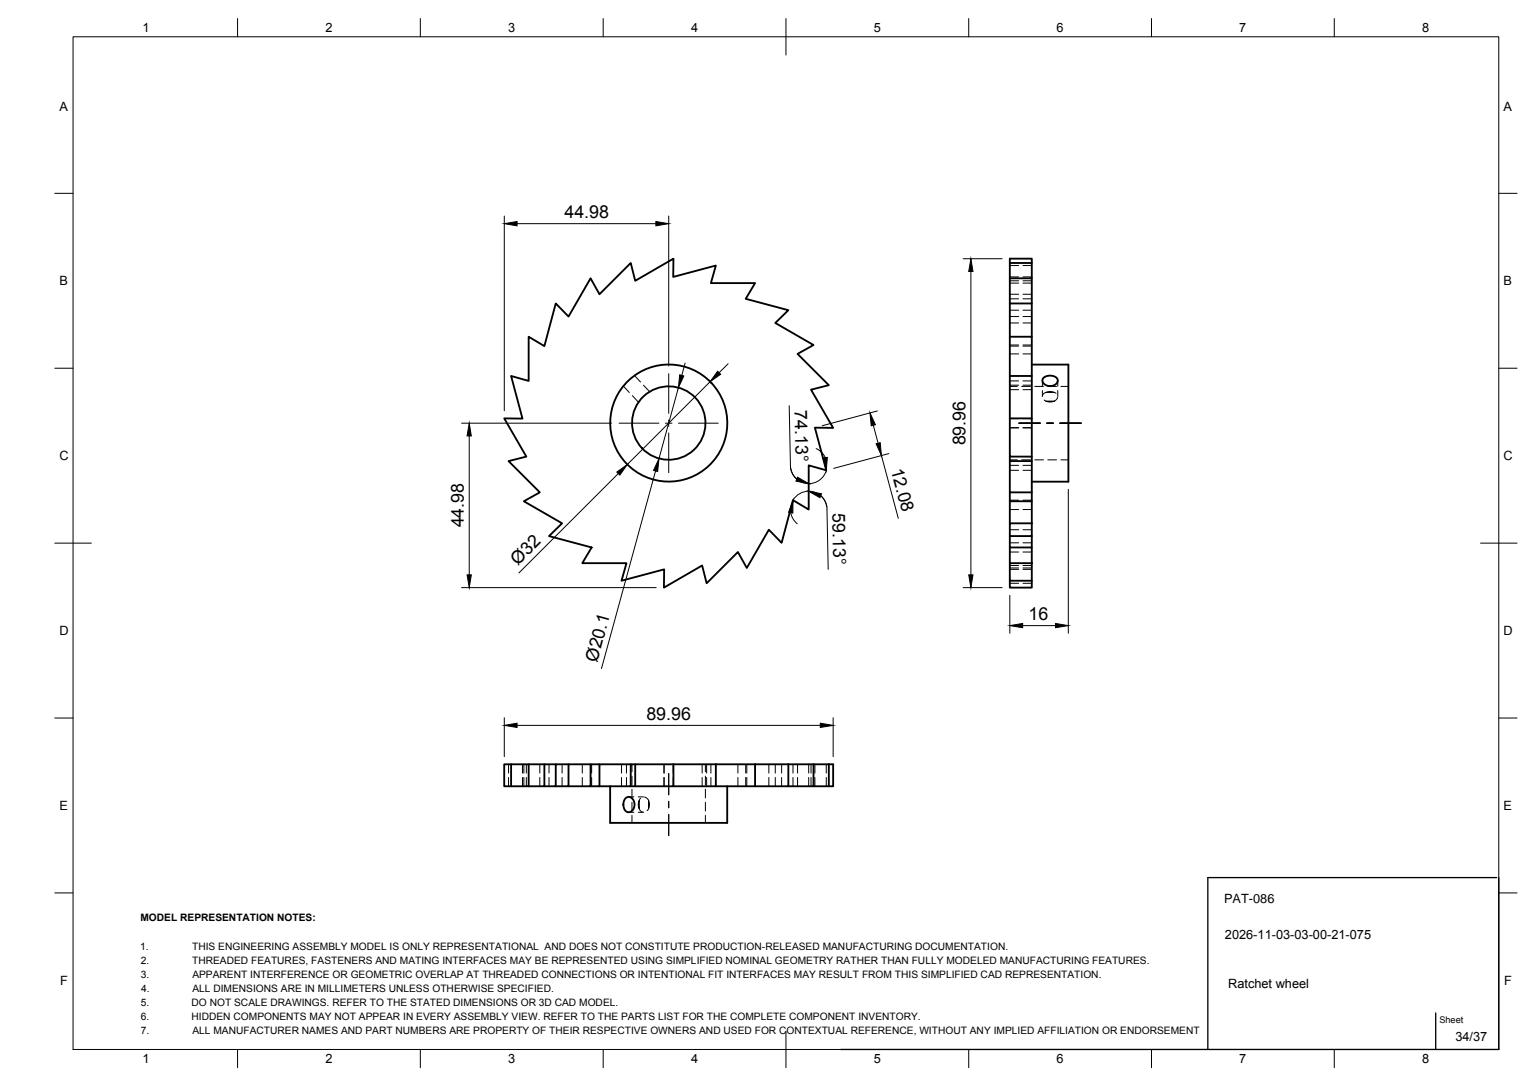
ISO-10303-21;
HEADER;
/* Generated by software containing ST-Developer
 * from STEP Tools, Inc. (www.steptools.com) 
 */

FILE_DESCRIPTION(
/* description */ ('Ratchet and pawl hand winch drum'),
/* implementation_level */ '2;1');

FILE_NAME(
/* name */ 'Ratchet wheel.step',
/* time_stamp */ '2026-10-27T12:42:58-07:00',
/* author */ (''),
/* organization */ (''),
/* preprocessor_version */ 'ST-DEVELOPER v20.2',
/* originating_system */ 'Autodesk Translation Framework v15.17.0.0',
/* authorisation */ '');

FILE_SCHEMA (('AUTOMOTIVE_DESIGN { 1 0 10303 214 3 1 1 }'));
ENDSEC;

DATA;
#10=MECHANICAL_DESIGN_GEOMETRIC_PRESENTATION_REPRESENTATION('',(#418),#11801);
#313=B_SPLINE_CURVE_WITH_KNOTS('',3,(#11023,#11024,#11025,#11026,#11027,
#11028,#11029,#11030,#11031,#11032,#11033,#11034,#11035,#11036),
 .UNSPECIFIED.,.F.,.F.,(4,2,2,2,2,2,4),(0.75600573798702,0.793568827564647,
0.872922520054201,0.952276212543756,1.03162990503331,1.11098359752287,1.14854668710049),
 .UNSPECIFIED.);
#314=B_SPLINE_CURVE_WITH_KNOTS('',3,(#11042,#11043,#11044,#11045,#11046,
#11047,#11048,#11049,#11050,#11051,#11052,#11053,#11054,#11055,#11056,#11057,
#11058,#11059),.UNSPECIFIED.,.F.,.F.,(4,2,2,2,2,2,2,2,4),(0.,0.0792028026112439,
0.158405605222488,0.237607602356377,0.316809599490267,0.396011596624156,
0.475213593758045,0.554416396369289,0.633619198980533),.UNSPECIFIED.);
#315=B_SPLINE_CURVE_WITH_KNOTS('',3,(#11060,#11061,#11062,#11063,#11064,
#11065,#11066,#11067,#11068,#11069,#11070,#11071,#11072,#11073,#11074,#11075,
#11076,#11077),.UNSPECIFIED.,.F.,.F.,(4,2,2,2,2,2,2,2,4),(0.633619198980533,
0.712822001591777,0.792024804203021,0.87122680133691,0.950428798470799,
1.02963079560469,1.10883279273858,1.18803559534982,1.26723839796107),
 .UNSPECIFIED.);
#316=B_SPLINE_CURVE_WITH_KNOTS('',3,(#11080,#11081,#11082,#11083,#11084,
#11085,#11086,#11087,#11088,#11089,#11090,#11091,#11092,#11093),
 .UNSPECIFIED.,.F.,.F.,(4,2,2,2,2,2,4),(0.121154929624516,0.158718019202143,
0.238071711691697,0.317425404181252,0.396779096670807,0.476132789160362,
0.513695878737989),.UNSPECIFIED.);
#349=SHAPE_REPRESENTATION_RELATIONSHIP('SRR','None',#11977,#383);
#383=ADVANCED_BREP_SHAPE_REPRESENTATION('',(#451),#11794);
#418=STYLED_ITEM('',(#12206),#451);
#451=MANIFOLD_SOLID_BREP('Body1',#6297);
#586=FACE_BOUND('',#1576,.T.);
#587=FACE_BOUND('',#1578,.T.);
#588=FACE_BOUND('',#1580,.T.);
#589=FACE_BOUND('',#1630,.T.);
#590=FACE_BOUND('',#1632,.T.);
#750=PLANE('',#7144);
#751=PLANE('',#7149);
#752=PLANE('',#7153);
#753=PLANE('',#7157);
#754=PLANE('',#7158);
#755=PLANE('',#7159);
#756=PLANE('',#7160);
#757=PLANE('',#7161);
#758=PLANE('',#7162);
#759=PLANE('',#7163);
#760=PLANE('',#7164);
#761=PLANE('',#7165);
#762=PLANE('',#7166);
#763=PLANE('',#7167);
#764=PLANE('',#7168);
#765=PLANE('',#7169);
#766=PLANE('',#7170);
#767=PLANE('',#7171);
#768=PLANE('',#7172);
#769=PLANE('',#7173);
#770=PLANE('',#7174);
#771=PLANE('',#7175);
#772=PLANE('',#7176);
#773=PLANE('',#7177);
#774=PLANE('',#7178);
#775=PLANE('',#7179);
#776=PLANE('',#7180);
#777=PLANE('',#7181);
#778=PLANE('',#7182);
#779=PLANE('',#7183);
#780=PLANE('',#7184);
#781=PLANE('',#7185);
#782=PLANE('',#7186);
#783=PLANE('',#7187);
#784=PLANE('',#7188);
#785=PLANE('',#7189);
#786=PLANE('',#7190);
#787=PLANE('',#7191);
#788=PLANE('',#7192);
#789=PLANE('',#7193);
#790=PLANE('',#7194);
#791=PLANE('',#7195);
#792=PLANE('',#7196);
#793=PLANE('',#7197);
#794=PLANE('',#7198);
#795=PLANE('',#7199);
#796=PLANE('',#7200);
#797=PLANE('',#7201);
#798=PLANE('',#7202);
#799=PLANE('',#7203);
#800=PLANE('',#7204);
#801=PLANE('',#7205);
#802=PLANE('',#7206);
#1086=FACE_OUTER_BOUND('',#1572,.T.);
#1087=FACE_OUTER_BOUND('',#1573,.T.);
#1088=FACE_OUTER_BOUND('',#1574,.T.);
#1089=FACE_OUTER_BOUND('',#1575,.T.);
#1090=FACE_OUTER_BOUND('',#1577,.T.);
#1091=FACE_OUTER_BOUND('',#1579,.T.);
#1092=FACE_OUTER_BOUND('',#1581,.T.);
#1093=FACE_OUTER_BOUND('',#1582,.T.);
#1094=FACE_OUTER_BOUND('',#1583,.T.);
#1095=FACE_OUTER_BOUND('',#1584,.T.);
#1096=FACE_OUTER_BOUND('',#1585,.T.);
#1097=FACE_OUTER_BOUND('',#1586,.T.);
#1098=FACE_OUTER_BOUND('',#1587,.T.);
#1099=FACE_OUTER_BOUND('',#1588,.T.);
#1100=FACE_OUTER_BOUND('',#1589,.T.);
#1101=FACE_OUTER_BOUND('',#1590,.T.);
#1102=FACE_OUTER_BOUND('',#1591,.T.);
#1103=FACE_OUTER_BOUND('',#1592,.T.);
#1104=FACE_OUTER_BOUND('',#1593,.T.);
#1105=FACE_OUTER_BOUND('',#1594,.T.);
#1106=FACE_OUTER_BOUND('',#1595,.T.);
#1107=FACE_OUTER_BOUND('',#1596,.T.);
#1108=FACE_OUTER_BOUND('',#1597,.T.);
#1109=FACE_OUTER_BOUND('',#1598,.T.);
#1110=FACE_OUTER_BOUND('',#1599,.T.);
#1111=FACE_OUTER_BOUND('',#1600,.T.);
#1112=FACE_OUTER_BOUND('',#1601,.T.);
#1113=FACE_OUTER_BOUND('',#1602,.T.);
#1114=FACE_OUTER_BOUND('',#1603,.T.);
#1115=FACE_OUTER_BOUND('',#1604,.T.);
#1116=FACE_OUTER_BOUND('',#1605,.T.);
#1117=FACE_OUTER_BOUND('',#1606,.T.);
#1118=FACE_OUTER_BOUND('',#1607,.T.);
#1119=FACE_OUTER_BOUND('',#1608,.T.);
#1120=FACE_OUTER_BOUND('',#1609,.T.);
#1121=FACE_OUTER_BOUND('',#1610,.T.);
#1122=FACE_OUTER_BOUND('',#1611,.T.);
#1123=FACE_OUTER_BOUND('',#1612,.T.);
#1124=FACE_OUTER_BOUND('',#1613,.T.);
#1125=FACE_OUTER_BOUND('',#1614,.T.);
#1126=FACE_OUTER_BOUND('',#1615,.T.);
#1127=FACE_OUTER_BOUND('',#1616,.T.);
#1128=FACE_OUTER_BOUND('',#1617,.T.);
#1129=FACE_OUTER_BOUND('',#1618,.T.);
#1130=FACE_OUTER_BOUND('',#1619,.T.);
#1131=FACE_OUTER_BOUND('',#1620,.T.);
#1132=FACE_OUTER_BOUND('',#1621,.T.);
#1133=FACE_OUTER_BOUND('',#1622,.T.);
#1134=FACE_OUTER_BOUND('',#1623,.T.);
#1135=FACE_OUTER_BOUND('',#1624,.T.);
#1136=FACE_OUTER_BOUND('',#1625,.T.);
#1137=FACE_OUTER_BOUND('',#1626,.T.);
#1138=FACE_OUTER_BOUND('',#1627,.T.);
#1139=FACE_OUTER_BOUND('',#1628,.T.);
#1140=FACE_OUTER_BOUND('',#1629,.T.);
#1141=FACE_OUTER_BOUND('',#1631,.T.);
#1572=EDGE_LOOP('',(#5271,#5272));
#1573=EDGE_LOOP('',(#5273,#5274,#5275,#5276,#5277,#5278,#5279,#5280,#5281));
#1574=EDGE_LOOP('',(#5282,#5283,#5284));
#1575=EDGE_LOOP('',(#5285,#5286,#5287,#5288));
#1576=EDGE_LOOP('',(#5289,#5290));
#1577=EDGE_LOOP('',(#5291));
#1578=EDGE_LOOP('',(#5292));
#1579=EDGE_LOOP('',(#5293,#5294,#5295,#5296));
#1580=EDGE_LOOP('',(#5297,#5298,#5299,#5300));
#1581=EDGE_LOOP('',(#5301,#5302,#5303,#5304));
#1582=EDGE_LOOP('',(#5305,#5306,#5307,#5308));
#1583=EDGE_LOOP('',(#5309,#5310,#5311,#5312));
#1584=EDGE_LOOP('',(#5313,#5314,#5315,#5316));
#1585=EDGE_LOOP('',(#5317,#5318,#5319,#5320));
#1586=EDGE_LOOP('',(#5321,#5322,#5323,#5324));
#1587=EDGE_LOOP('',(#5325,#5326,#5327,#5328));
#1588=EDGE_LOOP('',(#5329,#5330,#5331,#5332));
#1589=EDGE_LOOP('',(#5333,#5334,#5335,#5336));
#1590=EDGE_LOOP('',(#5337,#5338,#5339,#5340));
#1591=EDGE_LOOP('',(#5341,#5342,#5343,#5344));
#1592=EDGE_LOOP('',(#5345,#5346,#5347,#5348));
#1593=EDGE_LOOP('',(#5349,#5350,#5351,#5352));
#1594=EDGE_LOOP('',(#5353,#5354,#5355,#5356));
#1595=EDGE_LOOP('',(#5357,#5358,#5359,#5360));
#1596=EDGE_LOOP('',(#5361,#5362,#5363,#5364));
#1597=EDGE_LOOP('',(#5365,#5366,#5367,#5368));
#1598=EDGE_LOOP('',(#5369,#5370,#5371,#5372));
#1599=EDGE_LOOP('',(#5373,#5374,#5375,#5376));
#1600=EDGE_LOOP('',(#5377,#5378,#5379,#5380));
#1601=EDGE_LOOP('',(#5381,#5382,#5383,#5384));
#1602=EDGE_LOOP('',(#5385,#5386,#5387,#5388));
#1603=EDGE_LOOP('',(#5389,#5390,#5391,#5392));
#1604=EDGE_LOOP('',(#5393,#5394,#5395,#5396));
#1605=EDGE_LOOP('',(#5397,#5398,#5399,#5400));
#1606=EDGE_LOOP('',(#5401,#5402,#5403,#5404));
#1607=EDGE_LOOP('',(#5405,#5406,#5407,#5408));
#1608=EDGE_LOOP('',(#5409,#5410,#5411,#5412));
#1609=EDGE_LOOP('',(#5413,#5414,#5415,#5416));
#1610=EDGE_LOOP('',(#5417,#5418,#5419,#5420));
#1611=EDGE_LOOP('',(#5421,#5422,#5423,#5424));
#1612=EDGE_LOOP('',(#5425,#5426,#5427,#5428));
#1613=EDGE_LOOP('',(#5429,#5430,#5431,#5432));
#1614=EDGE_LOOP('',(#5433,#5434,#5435,#5436));
#1615=EDGE_LOOP('',(#5437,#5438,#5439,#5440));
#1616=EDGE_LOOP('',(#5441,#5442,#5443,#5444));
#1617=EDGE_LOOP('',(#5445,#5446,#5447,#5448));
#1618=EDGE_LOOP('',(#5449,#5450,#5451,#5452));
#1619=EDGE_LOOP('',(#5453,#5454,#5455,#5456));
#1620=EDGE_LOOP('',(#5457,#5458,#5459,#5460));
#1621=EDGE_LOOP('',(#5461,#5462,#5463,#5464));
#1622=EDGE_LOOP('',(#5465,#5466,#5467,#5468));
#1623=EDGE_LOOP('',(#5469,#5470,#5471,#5472));
#1624=EDGE_LOOP('',(#5473,#5474,#5475,#5476));
#1625=EDGE_LOOP('',(#5477,#5478,#5479,#5480));
#1626=EDGE_LOOP('',(#5481,#5482,#5483,#5484));
#1627=EDGE_LOOP('',(#5485,#5486,#5487,#5488));
#1628=EDGE_LOOP('',(#5489,#5490,#5491,#5492));
#1629=EDGE_LOOP('',(#5493,#5494,#5495,#5496,#5497,#5498,#5499,#5500,#5501,
#5502,#5503,#5504,#5505,#5506,#5507,#5508,#5509,#5510,#5511,#5512,#5513,
#5514,#5515,#5516,#5517,#5518,#5519,#5520,#5521,#5522,#5523,#5524,#5525,
#5526,#5527,#5528,#5529,#5530,#5531,#5532,#5533,#5534,#5535,#5536,#5537,
#5538,#5539,#5540));
#1630=EDGE_LOOP('',(#5541));
#1631=EDGE_LOOP('',(#5542,#5543,#5544,#5545,#5546,#5547,#5548,#5549,#5550,
#5551,#5552,#5553,#5554,#5555,#5556,#5557,#5558,#5559,#5560,#5561,#5562,
#5563,#5564,#5565,#5566,#5567,#5568,#5569,#5570,#5571,#5572,#5573,#5574,
#5575,#5576,#5577,#5578,#5579,#5580,#5581,#5582,#5583,#5584,#5585,#5586,
#5587,#5588,#5589));
#1632=EDGE_LOOP('',(#5590));
#1985=LINE('',#11019,#2496);
#1986=LINE('',#11040,#2497);
#1987=LINE('',#11095,#2498);
#1988=LINE('',#11100,#2499);
#1989=LINE('',#11108,#2500);
#1990=LINE('',#11112,#2501);
#1991=LINE('',#11114,#2502);
#1992=LINE('',#11116,#2503);
#1993=LINE('',#11117,#2504);
#1994=LINE('',#11120,#2505);
#1995=LINE('',#11122,#2506);
#1996=LINE('',#11123,#2507);
#1997=LINE('',#11126,#2508);
#1998=LINE('',#11128,#2509);
#1999=LINE('',#11129,#2510);
#2000=LINE('',#11132,#2511);
#2001=LINE('',#11134,#2512);
#2002=LINE('',#11135,#2513);
#2003=LINE('',#11138,#2514);
#2004=LINE('',#11140,#2515);
#2005=LINE('',#11141,#2516);
#2006=LINE('',#11144,#2517);
#2007=LINE('',#11146,#2518);
#2008=LINE('',#11147,#2519);
#2009=LINE('',#11150,#2520);
#2010=LINE('',#11152,#2521);
#2011=LINE('',#11153,#2522);
#2012=LINE('',#11156,#2523);
#2013=LINE('',#11158,#2524);
#2014=LINE('',#11159,#2525);
#2015=LINE('',#11162,#2526);
#2016=LINE('',#11164,#2527);
#2017=LINE('',#11165,#2528);
#2018=LINE('',#11168,#2529);
#2019=LINE('',#11170,#2530);
#2020=LINE('',#11171,#2531);
#2021=LINE('',#11174,#2532);
#2022=LINE('',#11176,#2533);
#2023=LINE('',#11177,#2534);
#2024=LINE('',#11180,#2535);
#2025=LINE('',#11182,#2536);
#2026=LINE('',#11183,#2537);
#2027=LINE('',#11186,#2538);
#2028=LINE('',#11188,#2539);
#2029=LINE('',#11189,#2540);
#2030=LINE('',#11192,#2541);
#2031=LINE('',#11194,#2542);
#2032=LINE('',#11195,#2543);
#2033=LINE('',#11198,#2544);
#2034=LINE('',#11200,#2545);
#2035=LINE('',#11201,#2546);
#2036=LINE('',#11204,#2547);
#2037=LINE('',#11206,#2548);
#2038=LINE('',#11207,#2549);
#2039=LINE('',#11210,#2550);
#2040=LINE('',#11212,#2551);
#2041=LINE('',#11213,#2552);
#2042=LINE('',#11216,#2553);
#2043=LINE('',#11218,#2554);
#2044=LINE('',#11219,#2555);
#2045=LINE('',#11222,#2556);
#2046=LINE('',#11224,#2557);
#2047=LINE('',#11225,#2558);
#2048=LINE('',#11228,#2559);
#2049=LINE('',#11230,#2560);
#2050=LINE('',#11231,#2561);
#2051=LINE('',#11234,#2562);
#2052=LINE('',#11236,#2563);
#2053=LINE('',#11237,#2564);
#2054=LINE('',#11240,#2565);
#2055=LINE('',#11242,#2566);
#2056=LINE('',#11243,#2567);
#2057=LINE('',#11246,#2568);
#2058=LINE('',#11248,#2569);
#2059=LINE('',#11249,#2570);
#2060=LINE('',#11252,#2571);
#2061=LINE('',#11254,#2572);
#2062=LINE('',#11255,#2573);
#2063=LINE('',#11258,#2574);
#2064=LINE('',#11260,#2575);
#2065=LINE('',#11261,#2576);
#2066=LINE('',#11264,#2577);
#2067=LINE('',#11266,#2578);
#2068=LINE('',#11267,#2579);
#2069=LINE('',#11270,#2580);
#2070=LINE('',#11272,#2581);
#2071=LINE('',#11273,#2582);
#2072=LINE('',#11276,#2583);
#2073=LINE('',#11278,#2584);
#2074=LINE('',#11279,#2585);
#2075=LINE('',#11282,#2586);
#2076=LINE('',#11284,#2587);
#2077=LINE('',#11285,#2588);
#2078=LINE('',#11288,#2589);
#2079=LINE('',#11290,#2590);
#2080=LINE('',#11291,#2591);
#2081=LINE('',#11294,#2592);
#2082=LINE('',#11296,#2593);
#2083=LINE('',#11297,#2594);
#2084=LINE('',#11300,#2595);
#2085=LINE('',#11302,#2596);
#2086=LINE('',#11303,#2597);
#2087=LINE('',#11306,#2598);
#2088=LINE('',#11308,#2599);
#2089=LINE('',#11309,#2600);
#2090=LINE('',#11312,#2601);
#2091=LINE('',#11314,#2602);
#2092=LINE('',#11315,#2603);
#2093=LINE('',#11318,#2604);
#2094=LINE('',#11320,#2605);
#2095=LINE('',#11321,#2606);
#2096=LINE('',#11324,#2607);
#2097=LINE('',#11326,#2608);
#2098=LINE('',#11327,#2609);
#2099=LINE('',#11330,#2610);
#2100=LINE('',#11332,#2611);
#2101=LINE('',#11333,#2612);
#2102=LINE('',#11336,#2613);
#2103=LINE('',#11338,#2614);
#2104=LINE('',#11339,#2615);
#2105=LINE('',#11342,#2616);
#2106=LINE('',#11344,#2617);
#2107=LINE('',#11345,#2618);
#2108=LINE('',#11348,#2619);
#2109=LINE('',#11350,#2620);
#2110=LINE('',#11351,#2621);
#2111=LINE('',#11354,#2622);
#2112=LINE('',#11356,#2623);
#2113=LINE('',#11357,#2624);
#2114=LINE('',#11360,#2625);
#2115=LINE('',#11362,#2626);
#2116=LINE('',#11363,#2627);
#2117=LINE('',#11366,#2628);
#2118=LINE('',#11368,#2629);
#2119=LINE('',#11369,#2630);
#2120=LINE('',#11372,#2631);
#2121=LINE('',#11374,#2632);
#2122=LINE('',#11375,#2633);
#2123=LINE('',#11378,#2634);
#2124=LINE('',#11380,#2635);
#2125=LINE('',#11381,#2636);
#2126=LINE('',#11384,#2637);
#2127=LINE('',#11386,#2638);
#2128=LINE('',#11387,#2639);
#2129=LINE('',#11390,#2640);
#2130=LINE('',#11392,#2641);
#2131=LINE('',#11393,#2642);
#2132=LINE('',#11395,#2643);
#2133=LINE('',#11396,#2644);
#2496=VECTOR('',#8578,1.);
#2497=VECTOR('',#8585,0.21);
#2498=VECTOR('',#8590,1.);
#2499=VECTOR('',#8595,1.6);
#2500=VECTOR('',#8606,1.005);
#2501=VECTOR('',#8609,1.);
#2502=VECTOR('',#8610,1.);
#2503=VECTOR('',#8611,1.);
#2504=VECTOR('',#8612,1.);
#2505=VECTOR('',#8615,1.);
#2506=VECTOR('',#8616,1.);
#2507=VECTOR('',#8617,1.);
#2508=VECTOR('',#8620,1.);
#2509=VECTOR('',#8621,1.);
#2510=VECTOR('',#8622,1.);
#2511=VECTOR('',#8625,1.);
#2512=VECTOR('',#8626,1.);
#2513=VECTOR('',#8627,1.);
#2514=VECTOR('',#8630,1.);
#2515=VECTOR('',#8631,1.);
#2516=VECTOR('',#8632,1.);
#2517=VECTOR('',#8635,1.);
#2518=VECTOR('',#8636,1.);
#2519=VECTOR('',#8637,1.);
#2520=VECTOR('',#8640,1.);
#2521=VECTOR('',#8641,1.);
#2522=VECTOR('',#8642,1.);
#2523=VECTOR('',#8645,1.);
#2524=VECTOR('',#8646,1.);
#2525=VECTOR('',#8647,1.);
#2526=VECTOR('',#8650,1.);
#2527=VECTOR('',#8651,1.);
#2528=VECTOR('',#8652,1.);
#2529=VECTOR('',#8655,1.);
#2530=VECTOR('',#8656,1.);
#2531=VECTOR('',#8657,1.);
#2532=VECTOR('',#8660,1.);
#2533=VECTOR('',#8661,1.);
#2534=VECTOR('',#8662,1.);
#2535=VECTOR('',#8665,1.);
#2536=VECTOR('',#8666,1.);
#2537=VECTOR('',#8667,1.);
#2538=VECTOR('',#8670,1.);
#2539=VECTOR('',#8671,1.);
#2540=VECTOR('',#8672,1.);
#2541=VECTOR('',#8675,1.);
#2542=VECTOR('',#8676,1.);
#2543=VECTOR('',#8677,1.);
#2544=VECTOR('',#8680,1.);
#2545=VECTOR('',#8681,1.);
#2546=VECTOR('',#8682,1.);
#2547=VECTOR('',#8685,1.);
#2548=VECTOR('',#8686,1.);
#2549=VECTOR('',#8687,1.);
#2550=VECTOR('',#8690,1.);
#2551=VECTOR('',#8691,1.);
#2552=VECTOR('',#8692,1.);
#2553=VECTOR('',#8695,1.);
#2554=VECTOR('',#8696,1.);
#2555=VECTOR('',#8697,1.);
#2556=VECTOR('',#8700,1.);
#2557=VECTOR('',#8701,1.);
#2558=VECTOR('',#8702,1.);
#2559=VECTOR('',#8705,1.);
#2560=VECTOR('',#8706,1.);
#2561=VECTOR('',#8707,1.);
#2562=VECTOR('',#8710,1.);
#2563=VECTOR('',#8711,1.);
#2564=VECTOR('',#8712,1.);
#2565=VECTOR('',#8715,1.);
#2566=VECTOR('',#8716,1.);
#2567=VECTOR('',#8717,1.);
#2568=VECTOR('',#8720,1.);
#2569=VECTOR('',#8721,1.);
#2570=VECTOR('',#8722,1.);
#2571=VECTOR('',#8725,1.);
#2572=VECTOR('',#8726,1.);
#2573=VECTOR('',#8727,1.);
#2574=VECTOR('',#8730,1.);
#2575=VECTOR('',#8731,1.);
#2576=VECTOR('',#8732,1.);
#2577=VECTOR('',#8735,1.);
#2578=VECTOR('',#8736,1.);
#2579=VECTOR('',#8737,1.);
#2580=VECTOR('',#8740,1.);
#2581=VECTOR('',#8741,1.);
#2582=VECTOR('',#8742,1.);
#2583=VECTOR('',#8745,1.);
#2584=VECTOR('',#8746,1.);
#2585=VECTOR('',#8747,1.);
#2586=VECTOR('',#8750,1.);
#2587=VECTOR('',#8751,1.);
#2588=VECTOR('',#8752,1.);
#2589=VECTOR('',#8755,1.);
#2590=VECTOR('',#8756,1.);
#2591=VECTOR('',#8757,1.);
#2592=VECTOR('',#8760,1.);
#2593=VECTOR('',#8761,1.);
#2594=VECTOR('',#8762,1.);
#2595=VECTOR('',#8765,1.);
#2596=VECTOR('',#8766,1.);
#2597=VECTOR('',#8767,1.);
#2598=VECTOR('',#8770,1.);
#2599=VECTOR('',#8771,1.);
#2600=VECTOR('',#8772,1.);
#2601=VECTOR('',#8775,1.);
#2602=VECTOR('',#8776,1.);
#2603=VECTOR('',#8777,1.);
#2604=VECTOR('',#8780,1.);
#2605=VECTOR('',#8781,1.);
#2606=VECTOR('',#8782,1.);
#2607=VECTOR('',#8785,1.);
#2608=VECTOR('',#8786,1.);
#2609=VECTOR('',#8787,1.);
#2610=VECTOR('',#8790,1.);
#2611=VECTOR('',#8791,1.);
#2612=VECTOR('',#8792,1.);
#2613=VECTOR('',#8795,1.);
#2614=VECTOR('',#8796,1.);
#2615=VECTOR('',#8797,1.);
#2616=VECTOR('',#8800,1.);
#2617=VECTOR('',#8801,1.);
#2618=VECTOR('',#8802,1.);
#2619=VECTOR('',#8805,1.);
#2620=VECTOR('',#8806,1.);
#2621=VECTOR('',#8807,1.);
#2622=VECTOR('',#8810,1.);
#2623=VECTOR('',#8811,1.);
#2624=VECTOR('',#8812,1.);
#2625=VECTOR('',#8815,1.);
#2626=VECTOR('',#8816,1.);
#2627=VECTOR('',#8817,1.);
#2628=VECTOR('',#8820,1.);
#2629=VECTOR('',#8821,1.);
#2630=VECTOR('',#8822,1.);
#2631=VECTOR('',#8825,1.);
#2632=VECTOR('',#8826,1.);
#2633=VECTOR('',#8827,1.);
#2634=VECTOR('',#8830,1.);
#2635=VECTOR('',#8831,1.);
#2636=VECTOR('',#8832,1.);
#2637=VECTOR('',#8835,1.);
#2638=VECTOR('',#8836,1.);
#2639=VECTOR('',#8837,1.);
#2640=VECTOR('',#8840,1.);
#2641=VECTOR('',#8841,1.);
#2642=VECTOR('',#8842,1.);
#2643=VECTOR('',#8845,1.);
#2644=VECTOR('',#8846,1.);
#2903=CIRCLE('',#7145,0.21);
#2904=CIRCLE('',#7147,0.21);
#2905=CIRCLE('',#7148,0.21);
#2906=CIRCLE('',#7151,1.6);
#2907=CIRCLE('',#7152,1.6);
#2908=CIRCLE('',#7154,1.005);
#2909=CIRCLE('',#7156,1.005);
#3290=VERTEX_POINT('',#11017);
#3291=VERTEX_POINT('',#11018);
#3292=VERTEX_POINT('',#11022);
#3293=VERTEX_POINT('',#11037);
#3294=VERTEX_POINT('',#11039);
#3295=VERTEX_POINT('',#11041);
#3296=VERTEX_POINT('',#11078);
#3297=VERTEX_POINT('',#11097);
#3298=VERTEX_POINT('',#11099);
#3299=VERTEX_POINT('',#11103);
#3300=VERTEX_POINT('',#11106);
#3301=VERTEX_POINT('',#11110);
#3302=VERTEX_POINT('',#11111);
#3303=VERTEX_POINT('',#11113);
#3304=VERTEX_POINT('',#11115);
#3305=VERTEX_POINT('',#11119);
#3306=VERTEX_POINT('',#11121);
#3307=VERTEX_POINT('',#11125);
#3308=VERTEX_POINT('',#11127);
#3309=VERTEX_POINT('',#11131);
#3310=VERTEX_POINT('',#11133);
#3311=VERTEX_POINT('',#11137);
#3312=VERTEX_POINT('',#11139);
#3313=VERTEX_POINT('',#11143);
#3314=VERTEX_POINT('',#11145);
#3315=VERTEX_POINT('',#11149);
#3316=VERTEX_POINT('',#11151);
#3317=VERTEX_POINT('',#11155);
#3318=VERTEX_POINT('',#11157);
#3319=VERTEX_POINT('',#11161);
#3320=VERTEX_POINT('',#11163);
#3321=VERTEX_POINT('',#11167);
#3322=VERTEX_POINT('',#11169);
#3323=VERTEX_POINT('',#11173);
#3324=VERTEX_POINT('',#11175);
#3325=VERTEX_POINT('',#11179);
#3326=VERTEX_POINT('',#11181);
#3327=VERTEX_POINT('',#11185);
#3328=VERTEX_POINT('',#11187);
#3329=VERTEX_POINT('',#11191);
#3330=VERTEX_POINT('',#11193);
#3331=VERTEX_POINT('',#11197);
#3332=VERTEX_POINT('',#11199);
#3333=VERTEX_POINT('',#11203);
#3334=VERTEX_POINT('',#11205);
#3335=VERTEX_POINT('',#11209);
#3336=VERTEX_POINT('',#11211);
#3337=VERTEX_POINT('',#11215);
#3338=VERTEX_POINT('',#11217);
#3339=VERTEX_POINT('',#11221);
#3340=VERTEX_POINT('',#11223);
#3341=VERTEX_POINT('',#11227);
#3342=VERTEX_POINT('',#11229);
#3343=VERTEX_POINT('',#11233);
#3344=VERTEX_POINT('',#11235);
#3345=VERTEX_POINT('',#11239);
#3346=VERTEX_POINT('',#11241);
#3347=VERTEX_POINT('',#11245);
#3348=VERTEX_POINT('',#11247);
#3349=VERTEX_POINT('',#11251);
#3350=VERTEX_POINT('',#11253);
#3351=VERTEX_POINT('',#11257);
#3352=VERTEX_POINT('',#11259);
#3353=VERTEX_POINT('',#11263);
#3354=VERTEX_POINT('',#11265);
#3355=VERTEX_POINT('',#11269);
#3356=VERTEX_POINT('',#11271);
#3357=VERTEX_POINT('',#11275);
#3358=VERTEX_POINT('',#11277);
#3359=VERTEX_POINT('',#11281);
#3360=VERTEX_POINT('',#11283);
#3361=VERTEX_POINT('',#11287);
#3362=VERTEX_POINT('',#11289);
#3363=VERTEX_POINT('',#11293);
#3364=VERTEX_POINT('',#11295);
#3365=VERTEX_POINT('',#11299);
#3366=VERTEX_POINT('',#11301);
#3367=VERTEX_POINT('',#11305);
#3368=VERTEX_POINT('',#11307);
#3369=VERTEX_POINT('',#11311);
#3370=VERTEX_POINT('',#11313);
#3371=VERTEX_POINT('',#11317);
#3372=VERTEX_POINT('',#11319);
#3373=VERTEX_POINT('',#11323);
#3374=VERTEX_POINT('',#11325);
#3375=VERTEX_POINT('',#11329);
#3376=VERTEX_POINT('',#11331);
#3377=VERTEX_POINT('',#11335);
#3378=VERTEX_POINT('',#11337);
#3379=VERTEX_POINT('',#11341);
#3380=VERTEX_POINT('',#11343);
#3381=VERTEX_POINT('',#11347);
#3382=VERTEX_POINT('',#11349);
#3383=VERTEX_POINT('',#11353);
#3384=VERTEX_POINT('',#11355);
#3385=VERTEX_POINT('',#11359);
#3386=VERTEX_POINT('',#11361);
#3387=VERTEX_POINT('',#11365);
#3388=VERTEX_POINT('',#11367);
#3389=VERTEX_POINT('',#11371);
#3390=VERTEX_POINT('',#11373);
#3391=VERTEX_POINT('',#11377);
#3392=VERTEX_POINT('',#11379);
#3393=VERTEX_POINT('',#11383);
#3394=VERTEX_POINT('',#11385);
#3395=VERTEX_POINT('',#11389);
#3396=VERTEX_POINT('',#11391);
#3979=EDGE_CURVE('',#3290,#3291,#1985,.T.);
#3980=EDGE_CURVE('',#3290,#3291,#2903,.T.);
#3981=EDGE_CURVE('',#3292,#3290,#313,.T.);
#3982=EDGE_CURVE('',#3293,#3292,#2904,.T.);
#3983=EDGE_CURVE('',#3293,#3294,#1986,.T.);
#3984=EDGE_CURVE('',#3295,#3294,#314,.T.);
#3985=EDGE_CURVE('',#3294,#3295,#315,.T.);
#3986=EDGE_CURVE('',#3296,#3293,#2905,.T.);
#3987=EDGE_CURVE('',#3291,#3296,#316,.T.);
#3988=EDGE_CURVE('',#3296,#3292,#1987,.T.);
#3989=EDGE_CURVE('',#3297,#3297,#2906,.T.);
#3990=EDGE_CURVE('',#3297,#3298,#1988,.T.);
#3991=EDGE_CURVE('',#3298,#3298,#2907,.T.);
#3992=EDGE_CURVE('',#3299,#3299,#2908,.T.);
#3993=EDGE_CURVE('',#3300,#3300,#2909,.T.);
#3994=EDGE_CURVE('',#3300,#3299,#1989,.T.);
#3995=EDGE_CURVE('',#3301,#3302,#1990,.T.);
#3996=EDGE_CURVE('',#3301,#3303,#1991,.T.);
#3997=EDGE_CURVE('',#3304,#3303,#1992,.T.);
#3998=EDGE_CURVE('',#3302,#3304,#1993,.T.);
#3999=EDGE_CURVE('',#3302,#3305,#1994,.T.);
#4000=EDGE_CURVE('',#3306,#3304,#1995,.T.);
#4001=EDGE_CURVE('',#3305,#3306,#1996,.T.);
#4002=EDGE_CURVE('',#3305,#3307,#1997,.T.);
#4003=EDGE_CURVE('',#3308,#3306,#1998,.T.);
#4004=EDGE_CURVE('',#3307,#3308,#1999,.T.);
#4005=EDGE_CURVE('',#3307,#3309,#2000,.T.);
#4006=EDGE_CURVE('',#3310,#3308,#2001,.T.);
#4007=EDGE_CURVE('',#3309,#3310,#2002,.T.);
#4008=EDGE_CURVE('',#3309,#3311,#2003,.T.);
#4009=EDGE_CURVE('',#3312,#3310,#2004,.T.);
#4010=EDGE_CURVE('',#3311,#3312,#2005,.T.);
#4011=EDGE_CURVE('',#3311,#3313,#2006,.T.);
#4012=EDGE_CURVE('',#3314,#3312,#2007,.T.);
#4013=EDGE_CURVE('',#3313,#3314,#2008,.T.);
#4014=EDGE_CURVE('',#3313,#3315,#2009,.T.);
#4015=EDGE_CURVE('',#3316,#3314,#2010,.T.);
#4016=EDGE_CURVE('',#3315,#3316,#2011,.T.);
#4017=EDGE_CURVE('',#3315,#3317,#2012,.T.);
#4018=EDGE_CURVE('',#3318,#3316,#2013,.T.);
#4019=EDGE_CURVE('',#3317,#3318,#2014,.T.);
#4020=EDGE_CURVE('',#3317,#3319,#2015,.T.);
#4021=EDGE_CURVE('',#3320,#3318,#2016,.T.);
#4022=EDGE_CURVE('',#3319,#3320,#2017,.T.);
#4023=EDGE_CURVE('',#3319,#3321,#2018,.T.);
#4024=EDGE_CURVE('',#3322,#3320,#2019,.T.);
#4025=EDGE_CURVE('',#3321,#3322,#2020,.T.);
#4026=EDGE_CURVE('',#3321,#3323,#2021,.T.);
#4027=EDGE_CURVE('',#3324,#3322,#2022,.T.);
#4028=EDGE_CURVE('',#3323,#3324,#2023,.T.);
#4029=EDGE_CURVE('',#3323,#3325,#2024,.T.);
#4030=EDGE_CURVE('',#3326,#3324,#2025,.T.);
#4031=EDGE_CURVE('',#3325,#3326,#2026,.T.);
#4032=EDGE_CURVE('',#3325,#3327,#2027,.T.);
#4033=EDGE_CURVE('',#3328,#3326,#2028,.T.);
#4034=EDGE_CURVE('',#3327,#3328,#2029,.T.);
#4035=EDGE_CURVE('',#3327,#3329,#2030,.T.);
#4036=EDGE_CURVE('',#3330,#3328,#2031,.T.);
#4037=EDGE_CURVE('',#3329,#3330,#2032,.T.);
#4038=EDGE_CURVE('',#3329,#3331,#2033,.T.);
#4039=EDGE_CURVE('',#3332,#3330,#2034,.T.);
#4040=EDGE_CURVE('',#3331,#3332,#2035,.T.);
#4041=EDGE_CURVE('',#3331,#3333,#2036,.T.);
#4042=EDGE_CURVE('',#3334,#3332,#2037,.T.);
#4043=EDGE_CURVE('',#3333,#3334,#2038,.T.);
#4044=EDGE_CURVE('',#3333,#3335,#2039,.T.);
#4045=EDGE_CURVE('',#3336,#3334,#2040,.T.);
#4046=EDGE_CURVE('',#3335,#3336,#2041,.T.);
#4047=EDGE_CURVE('',#3335,#3337,#2042,.T.);
#4048=EDGE_CURVE('',#3338,#3336,#2043,.T.);
#4049=EDGE_CURVE('',#3337,#3338,#2044,.T.);
#4050=EDGE_CURVE('',#3337,#3339,#2045,.T.);
#4051=EDGE_CURVE('',#3340,#3338,#2046,.T.);
#4052=EDGE_CURVE('',#3339,#3340,#2047,.T.);
#4053=EDGE_CURVE('',#3339,#3341,#2048,.T.);
#4054=EDGE_CURVE('',#3342,#3340,#2049,.T.);
#4055=EDGE_CURVE('',#3341,#3342,#2050,.T.);
#4056=EDGE_CURVE('',#3341,#3343,#2051,.T.);
#4057=EDGE_CURVE('',#3344,#3342,#2052,.T.);
#4058=EDGE_CURVE('',#3343,#3344,#2053,.T.);
#4059=EDGE_CURVE('',#3343,#3345,#2054,.T.);
#4060=EDGE_CURVE('',#3346,#3344,#2055,.T.);
#4061=EDGE_CURVE('',#3345,#3346,#2056,.T.);
#4062=EDGE_CURVE('',#3345,#3347,#2057,.T.);
#4063=EDGE_CURVE('',#3348,#3346,#2058,.T.);
#4064=EDGE_CURVE('',#3347,#3348,#2059,.T.);
#4065=EDGE_CURVE('',#3347,#3349,#2060,.T.);
#4066=EDGE_CURVE('',#3350,#3348,#2061,.T.);
#4067=EDGE_CURVE('',#3349,#3350,#2062,.T.);
#4068=EDGE_CURVE('',#3349,#3351,#2063,.T.);
#4069=EDGE_CURVE('',#3352,#3350,#2064,.T.);
#4070=EDGE_CURVE('',#3351,#3352,#2065,.T.);
#4071=EDGE_CURVE('',#3351,#3353,#2066,.T.);
#4072=EDGE_CURVE('',#3354,#3352,#2067,.T.);
#4073=EDGE_CURVE('',#3353,#3354,#2068,.T.);
#4074=EDGE_CURVE('',#3353,#3355,#2069,.T.);
#4075=EDGE_CURVE('',#3356,#3354,#2070,.T.);
#4076=EDGE_CURVE('',#3355,#3356,#2071,.T.);
#4077=EDGE_CURVE('',#3355,#3357,#2072,.T.);
#4078=EDGE_CURVE('',#3358,#3356,#2073,.T.);
#4079=EDGE_CURVE('',#3357,#3358,#2074,.T.);
#4080=EDGE_CURVE('',#3357,#3359,#2075,.T.);
#4081=EDGE_CURVE('',#3360,#3358,#2076,.T.);
#4082=EDGE_CURVE('',#3359,#3360,#2077,.T.);
#4083=EDGE_CURVE('',#3359,#3361,#2078,.T.);
#4084=EDGE_CURVE('',#3362,#3360,#2079,.T.);
#4085=EDGE_CURVE('',#3361,#3362,#2080,.T.);
#4086=EDGE_CURVE('',#3361,#3363,#2081,.T.);
#4087=EDGE_CURVE('',#3364,#3362,#2082,.T.);
#4088=EDGE_CURVE('',#3363,#3364,#2083,.T.);
#4089=EDGE_CURVE('',#3363,#3365,#2084,.T.);
#4090=EDGE_CURVE('',#3366,#3364,#2085,.T.);
#4091=EDGE_CURVE('',#3365,#3366,#2086,.T.);
#4092=EDGE_CURVE('',#3365,#3367,#2087,.T.);
#4093=EDGE_CURVE('',#3368,#3366,#2088,.T.);
#4094=EDGE_CURVE('',#3367,#3368,#2089,.T.);
#4095=EDGE_CURVE('',#3367,#3369,#2090,.T.);
#4096=EDGE_CURVE('',#3370,#3368,#2091,.T.);
#4097=EDGE_CURVE('',#3369,#3370,#2092,.T.);
#4098=EDGE_CURVE('',#3369,#3371,#2093,.T.);
#4099=EDGE_CURVE('',#3372,#3370,#2094,.T.);
#4100=EDGE_CURVE('',#3371,#3372,#2095,.T.);
#4101=EDGE_CURVE('',#3371,#3373,#2096,.T.);
#4102=EDGE_CURVE('',#3374,#3372,#2097,.T.);
#4103=EDGE_CURVE('',#3373,#3374,#2098,.T.);
#4104=EDGE_CURVE('',#3373,#3375,#2099,.T.);
#4105=EDGE_CURVE('',#3376,#3374,#2100,.T.);
#4106=EDGE_CURVE('',#3375,#3376,#2101,.T.);
#4107=EDGE_CURVE('',#3375,#3377,#2102,.T.);
#4108=EDGE_CURVE('',#3378,#3376,#2103,.T.);
#4109=EDGE_CURVE('',#3377,#3378,#2104,.T.);
#4110=EDGE_CURVE('',#3377,#3379,#2105,.T.);
#4111=EDGE_CURVE('',#3380,#3378,#2106,.T.);
#4112=EDGE_CURVE('',#3379,#3380,#2107,.T.);
#4113=EDGE_CURVE('',#3379,#3381,#2108,.T.);
#4114=EDGE_CURVE('',#3382,#3380,#2109,.T.);
#4115=EDGE_CURVE('',#3381,#3382,#2110,.T.);
#4116=EDGE_CURVE('',#3381,#3383,#2111,.T.);
#4117=EDGE_CURVE('',#3384,#3382,#2112,.T.);
#4118=EDGE_CURVE('',#3383,#3384,#2113,.T.);
#4119=EDGE_CURVE('',#3383,#3385,#2114,.T.);
#4120=EDGE_CURVE('',#3386,#3384,#2115,.T.);
#4121=EDGE_CURVE('',#3385,#3386,#2116,.T.);
#4122=EDGE_CURVE('',#3385,#3387,#2117,.T.);
#4123=EDGE_CURVE('',#3388,#3386,#2118,.T.);
#4124=EDGE_CURVE('',#3387,#3388,#2119,.T.);
#4125=EDGE_CURVE('',#3387,#3389,#2120,.T.);
#4126=EDGE_CURVE('',#3390,#3388,#2121,.T.);
#4127=EDGE_CURVE('',#3389,#3390,#2122,.T.);
#4128=EDGE_CURVE('',#3389,#3391,#2123,.T.);
#4129=EDGE_CURVE('',#3392,#3390,#2124,.T.);
#4130=EDGE_CURVE('',#3391,#3392,#2125,.T.);
#4131=EDGE_CURVE('',#3391,#3393,#2126,.T.);
#4132=EDGE_CURVE('',#3394,#3392,#2127,.T.);
#4133=EDGE_CURVE('',#3393,#3394,#2128,.T.);
#4134=EDGE_CURVE('',#3393,#3395,#2129,.T.);
#4135=EDGE_CURVE('',#3396,#3394,#2130,.T.);
#4136=EDGE_CURVE('',#3395,#3396,#2131,.T.);
#4137=EDGE_CURVE('',#3395,#3301,#2132,.T.);
#4138=EDGE_CURVE('',#3303,#3396,#2133,.T.);
#5271=ORIENTED_EDGE('',*,*,#3979,.F.);
#5272=ORIENTED_EDGE('',*,*,#3980,.T.);
#5273=ORIENTED_EDGE('',*,*,#3981,.F.);
#5274=ORIENTED_EDGE('',*,*,#3982,.F.);
#5275=ORIENTED_EDGE('',*,*,#3983,.T.);
#5276=ORIENTED_EDGE('',*,*,#3984,.F.);
#5277=ORIENTED_EDGE('',*,*,#3985,.F.);
#5278=ORIENTED_EDGE('',*,*,#3983,.F.);
#5279=ORIENTED_EDGE('',*,*,#3986,.F.);
#5280=ORIENTED_EDGE('',*,*,#3987,.F.);
#5281=ORIENTED_EDGE('',*,*,#3980,.F.);
#5282=ORIENTED_EDGE('',*,*,#3988,.F.);
#5283=ORIENTED_EDGE('',*,*,#3986,.T.);
#5284=ORIENTED_EDGE('',*,*,#3982,.T.);
#5285=ORIENTED_EDGE('',*,*,#3989,.F.);
#5286=ORIENTED_EDGE('',*,*,#3990,.T.);
#5287=ORIENTED_EDGE('',*,*,#3991,.F.);
#5288=ORIENTED_EDGE('',*,*,#3990,.F.);
#5289=ORIENTED_EDGE('',*,*,#3984,.T.);
#5290=ORIENTED_EDGE('',*,*,#3985,.T.);
#5291=ORIENTED_EDGE('',*,*,#3989,.T.);
#5292=ORIENTED_EDGE('',*,*,#3992,.T.);
#5293=ORIENTED_EDGE('',*,*,#3993,.F.);
#5294=ORIENTED_EDGE('',*,*,#3994,.T.);
#5295=ORIENTED_EDGE('',*,*,#3992,.F.);
#5296=ORIENTED_EDGE('',*,*,#3994,.F.);
#5297=ORIENTED_EDGE('',*,*,#3987,.T.);
#5298=ORIENTED_EDGE('',*,*,#3988,.T.);
#5299=ORIENTED_EDGE('',*,*,#3981,.T.);
#5300=ORIENTED_EDGE('',*,*,#3979,.T.);
#5301=ORIENTED_EDGE('',*,*,#3995,.F.);
#5302=ORIENTED_EDGE('',*,*,#3996,.T.);
#5303=ORIENTED_EDGE('',*,*,#3997,.F.);
#5304=ORIENTED_EDGE('',*,*,#3998,.F.);
#5305=ORIENTED_EDGE('',*,*,#3999,.F.);
#5306=ORIENTED_EDGE('',*,*,#3998,.T.);
#5307=ORIENTED_EDGE('',*,*,#4000,.F.);
#5308=ORIENTED_EDGE('',*,*,#4001,.F.);
#5309=ORIENTED_EDGE('',*,*,#4002,.F.);
#5310=ORIENTED_EDGE('',*,*,#4001,.T.);
#5311=ORIENTED_EDGE('',*,*,#4003,.F.);
#5312=ORIENTED_EDGE('',*,*,#4004,.F.);
#5313=ORIENTED_EDGE('',*,*,#4005,.F.);
#5314=ORIENTED_EDGE('',*,*,#4004,.T.);
#5315=ORIENTED_EDGE('',*,*,#4006,.F.);
#5316=ORIENTED_EDGE('',*,*,#4007,.F.);
#5317=ORIENTED_EDGE('',*,*,#4008,.F.);
#5318=ORIENTED_EDGE('',*,*,#4007,.T.);
#5319=ORIENTED_EDGE('',*,*,#4009,.F.);
#5320=ORIENTED_EDGE('',*,*,#4010,.F.);
#5321=ORIENTED_EDGE('',*,*,#4011,.F.);
#5322=ORIENTED_EDGE('',*,*,#4010,.T.);
#5323=ORIENTED_EDGE('',*,*,#4012,.F.);
#5324=ORIENTED_EDGE('',*,*,#4013,.F.);
#5325=ORIENTED_EDGE('',*,*,#4014,.F.);
#5326=ORIENTED_EDGE('',*,*,#4013,.T.);
#5327=ORIENTED_EDGE('',*,*,#4015,.F.);
#5328=ORIENTED_EDGE('',*,*,#4016,.F.);
#5329=ORIENTED_EDGE('',*,*,#4017,.F.);
#5330=ORIENTED_EDGE('',*,*,#4016,.T.);
#5331=ORIENTED_EDGE('',*,*,#4018,.F.);
#5332=ORIENTED_EDGE('',*,*,#4019,.F.);
#5333=ORIENTED_EDGE('',*,*,#4020,.F.);
#5334=ORIENTED_EDGE('',*,*,#4019,.T.);
#5335=ORIENTED_EDGE('',*,*,#4021,.F.);
#5336=ORIENTED_EDGE('',*,*,#4022,.F.);
#5337=ORIENTED_EDGE('',*,*,#4023,.F.);
#5338=ORIENTED_EDGE('',*,*,#4022,.T.);
#5339=ORIENTED_EDGE('',*,*,#4024,.F.);
#5340=ORIENTED_EDGE('',*,*,#4025,.F.);
#5341=ORIENTED_EDGE('',*,*,#4026,.F.);
#5342=ORIENTED_EDGE('',*,*,#4025,.T.);
#5343=ORIENTED_EDGE('',*,*,#4027,.F.);
#5344=ORIENTED_EDGE('',*,*,#4028,.F.);
#5345=ORIENTED_EDGE('',*,*,#4029,.F.);
#5346=ORIENTED_EDGE('',*,*,#4028,.T.);
#5347=ORIENTED_EDGE('',*,*,#4030,.F.);
#5348=ORIENTED_EDGE('',*,*,#4031,.F.);
#5349=ORIENTED_EDGE('',*,*,#4032,.F.);
#5350=ORIENTED_EDGE('',*,*,#4031,.T.);
#5351=ORIENTED_EDGE('',*,*,#4033,.F.);
#5352=ORIENTED_EDGE('',*,*,#4034,.F.);
#5353=ORIENTED_EDGE('',*,*,#4035,.F.);
#5354=ORIENTED_EDGE('',*,*,#4034,.T.);
#5355=ORIENTED_EDGE('',*,*,#4036,.F.);
#5356=ORIENTED_EDGE('',*,*,#4037,.F.);
#5357=ORIENTED_EDGE('',*,*,#4038,.F.);
#5358=ORIENTED_EDGE('',*,*,#4037,.T.);
#5359=ORIENTED_EDGE('',*,*,#4039,.F.);
#5360=ORIENTED_EDGE('',*,*,#4040,.F.);
#5361=ORIENTED_EDGE('',*,*,#4041,.F.);
#5362=ORIENTED_EDGE('',*,*,#4040,.T.);
#5363=ORIENTED_EDGE('',*,*,#4042,.F.);
#5364=ORIENTED_EDGE('',*,*,#4043,.F.);
#5365=ORIENTED_EDGE('',*,*,#4044,.F.);
#5366=ORIENTED_EDGE('',*,*,#4043,.T.);
#5367=ORIENTED_EDGE('',*,*,#4045,.F.);
#5368=ORIENTED_EDGE('',*,*,#4046,.F.);
#5369=ORIENTED_EDGE('',*,*,#4047,.F.);
#5370=ORIENTED_EDGE('',*,*,#4046,.T.);
#5371=ORIENTED_EDGE('',*,*,#4048,.F.);
#5372=ORIENTED_EDGE('',*,*,#4049,.F.);
#5373=ORIENTED_EDGE('',*,*,#4050,.F.);
#5374=ORIENTED_EDGE('',*,*,#4049,.T.);
#5375=ORIENTED_EDGE('',*,*,#4051,.F.);
#5376=ORIENTED_EDGE('',*,*,#4052,.F.);
#5377=ORIENTED_EDGE('',*,*,#4053,.F.);
#5378=ORIENTED_EDGE('',*,*,#4052,.T.);
#5379=ORIENTED_EDGE('',*,*,#4054,.F.);
#5380=ORIENTED_EDGE('',*,*,#4055,.F.);
#5381=ORIENTED_EDGE('',*,*,#4056,.F.);
#5382=ORIENTED_EDGE('',*,*,#4055,.T.);
#5383=ORIENTED_EDGE('',*,*,#4057,.F.);
#5384=ORIENTED_EDGE('',*,*,#4058,.F.);
#5385=ORIENTED_EDGE('',*,*,#4059,.F.);
#5386=ORIENTED_EDGE('',*,*,#4058,.T.);
#5387=ORIENTED_EDGE('',*,*,#4060,.F.);
#5388=ORIENTED_EDGE('',*,*,#4061,.F.);
#5389=ORIENTED_EDGE('',*,*,#4062,.F.);
#5390=ORIENTED_EDGE('',*,*,#4061,.T.);
#5391=ORIENTED_EDGE('',*,*,#4063,.F.);
#5392=ORIENTED_EDGE('',*,*,#4064,.F.);
#5393=ORIENTED_EDGE('',*,*,#4065,.F.);
#5394=ORIENTED_EDGE('',*,*,#4064,.T.);
#5395=ORIENTED_EDGE('',*,*,#4066,.F.);
#5396=ORIENTED_EDGE('',*,*,#4067,.F.);
#5397=ORIENTED_EDGE('',*,*,#4068,.F.);
#5398=ORIENTED_EDGE('',*,*,#4067,.T.);
#5399=ORIENTED_EDGE('',*,*,#4069,.F.);
#5400=ORIENTED_EDGE('',*,*,#4070,.F.);
#5401=ORIENTED_EDGE('',*,*,#4071,.F.);
#5402=ORIENTED_EDGE('',*,*,#4070,.T.);
#5403=ORIENTED_EDGE('',*,*,#4072,.F.);
#5404=ORIENTED_EDGE('',*,*,#4073,.F.);
#5405=ORIENTED_EDGE('',*,*,#4074,.F.);
#5406=ORIENTED_EDGE('',*,*,#4073,.T.);
#5407=ORIENTED_EDGE('',*,*,#4075,.F.);
#5408=ORIENTED_EDGE('',*,*,#4076,.F.);
#5409=ORIENTED_EDGE('',*,*,#4077,.F.);
#5410=ORIENTED_EDGE('',*,*,#4076,.T.);
#5411=ORIENTED_EDGE('',*,*,#4078,.F.);
#5412=ORIENTED_EDGE('',*,*,#4079,.F.);
#5413=ORIENTED_EDGE('',*,*,#4080,.F.);
#5414=ORIENTED_EDGE('',*,*,#4079,.T.);
#5415=ORIENTED_EDGE('',*,*,#4081,.F.);
#5416=ORIENTED_EDGE('',*,*,#4082,.F.);
#5417=ORIENTED_EDGE('',*,*,#4083,.F.);
#5418=ORIENTED_EDGE('',*,*,#4082,.T.);
#5419=ORIENTED_EDGE('',*,*,#4084,.F.);
#5420=ORIENTED_EDGE('',*,*,#4085,.F.);
#5421=ORIENTED_EDGE('',*,*,#4086,.F.);
#5422=ORIENTED_EDGE('',*,*,#4085,.T.);
#5423=ORIENTED_EDGE('',*,*,#4087,.F.);
#5424=ORIENTED_EDGE('',*,*,#4088,.F.);
#5425=ORIENTED_EDGE('',*,*,#4089,.F.);
#5426=ORIENTED_EDGE('',*,*,#4088,.T.);
#5427=ORIENTED_EDGE('',*,*,#4090,.F.);
#5428=ORIENTED_EDGE('',*,*,#4091,.F.);
#5429=ORIENTED_EDGE('',*,*,#4092,.F.);
#5430=ORIENTED_EDGE('',*,*,#4091,.T.);
#5431=ORIENTED_EDGE('',*,*,#4093,.F.);
#5432=ORIENTED_EDGE('',*,*,#4094,.F.);
#5433=ORIENTED_EDGE('',*,*,#4095,.F.);
#5434=ORIENTED_EDGE('',*,*,#4094,.T.);
#5435=ORIENTED_EDGE('',*,*,#4096,.F.);
#5436=ORIENTED_EDGE('',*,*,#4097,.F.);
#5437=ORIENTED_EDGE('',*,*,#4098,.F.);
#5438=ORIENTED_EDGE('',*,*,#4097,.T.);
#5439=ORIENTED_EDGE('',*,*,#4099,.F.);
#5440=ORIENTED_EDGE('',*,*,#4100,.F.);
#5441=ORIENTED_EDGE('',*,*,#4101,.F.);
#5442=ORIENTED_EDGE('',*,*,#4100,.T.);
#5443=ORIENTED_EDGE('',*,*,#4102,.F.);
#5444=ORIENTED_EDGE('',*,*,#4103,.F.);
#5445=ORIENTED_EDGE('',*,*,#4104,.F.);
#5446=ORIENTED_EDGE('',*,*,#4103,.T.);
#5447=ORIENTED_EDGE('',*,*,#4105,.F.);
#5448=ORIENTED_EDGE('',*,*,#4106,.F.);
#5449=ORIENTED_EDGE('',*,*,#4107,.F.);
#5450=ORIENTED_EDGE('',*,*,#4106,.T.);
#5451=ORIENTED_EDGE('',*,*,#4108,.F.);
#5452=ORIENTED_EDGE('',*,*,#4109,.F.);
#5453=ORIENTED_EDGE('',*,*,#4110,.F.);
#5454=ORIENTED_EDGE('',*,*,#4109,.T.);
#5455=ORIENTED_EDGE('',*,*,#4111,.F.);
#5456=ORIENTED_EDGE('',*,*,#4112,.F.);
#5457=ORIENTED_EDGE('',*,*,#4113,.F.);
#5458=ORIENTED_EDGE('',*,*,#4112,.T.);
#5459=ORIENTED_EDGE('',*,*,#4114,.F.);
#5460=ORIENTED_EDGE('',*,*,#4115,.F.);
#5461=ORIENTED_EDGE('',*,*,#4116,.F.);
#5462=ORIENTED_EDGE('',*,*,#4115,.T.);
#5463=ORIENTED_EDGE('',*,*,#4117,.F.);
#5464=ORIENTED_EDGE('',*,*,#4118,.F.);
#5465=ORIENTED_EDGE('',*,*,#4119,.F.);
#5466=ORIENTED_EDGE('',*,*,#4118,.T.);
#5467=ORIENTED_EDGE('',*,*,#4120,.F.);
#5468=ORIENTED_EDGE('',*,*,#4121,.F.);
#5469=ORIENTED_EDGE('',*,*,#4122,.F.);
#5470=ORIENTED_EDGE('',*,*,#4121,.T.);
#5471=ORIENTED_EDGE('',*,*,#4123,.F.);
#5472=ORIENTED_EDGE('',*,*,#4124,.F.);
#5473=ORIENTED_EDGE('',*,*,#4125,.F.);
#5474=ORIENTED_EDGE('',*,*,#4124,.T.);
#5475=ORIENTED_EDGE('',*,*,#4126,.F.);
#5476=ORIENTED_EDGE('',*,*,#4127,.F.);
#5477=ORIENTED_EDGE('',*,*,#4128,.F.);
#5478=ORIENTED_EDGE('',*,*,#4127,.T.);
#5479=ORIENTED_EDGE('',*,*,#4129,.F.);
#5480=ORIENTED_EDGE('',*,*,#4130,.F.);
#5481=ORIENTED_EDGE('',*,*,#4131,.F.);
#5482=ORIENTED_EDGE('',*,*,#4130,.T.);
#5483=ORIENTED_EDGE('',*,*,#4132,.F.);
#5484=ORIENTED_EDGE('',*,*,#4133,.F.);
#5485=ORIENTED_EDGE('',*,*,#4134,.F.);
#5486=ORIENTED_EDGE('',*,*,#4133,.T.);
#5487=ORIENTED_EDGE('',*,*,#4135,.F.);
#5488=ORIENTED_EDGE('',*,*,#4136,.F.);
#5489=ORIENTED_EDGE('',*,*,#4137,.F.);
#5490=ORIENTED_EDGE('',*,*,#4136,.T.);
#5491=ORIENTED_EDGE('',*,*,#4138,.F.);
#5492=ORIENTED_EDGE('',*,*,#3996,.F.);
#5493=ORIENTED_EDGE('',*,*,#4138,.T.);
#5494=ORIENTED_EDGE('',*,*,#4135,.T.);
#5495=ORIENTED_EDGE('',*,*,#4132,.T.);
#5496=ORIENTED_EDGE('',*,*,#4129,.T.);
#5497=ORIENTED_EDGE('',*,*,#4126,.T.);
#5498=ORIENTED_EDGE('',*,*,#4123,.T.);
#5499=ORIENTED_EDGE('',*,*,#4120,.T.);
#5500=ORIENTED_EDGE('',*,*,#4117,.T.);
#5501=ORIENTED_EDGE('',*,*,#4114,.T.);
#5502=ORIENTED_EDGE('',*,*,#4111,.T.);
#5503=ORIENTED_EDGE('',*,*,#4108,.T.);
#5504=ORIENTED_EDGE('',*,*,#4105,.T.);
#5505=ORIENTED_EDGE('',*,*,#4102,.T.);
#5506=ORIENTED_EDGE('',*,*,#4099,.T.);
#5507=ORIENTED_EDGE('',*,*,#4096,.T.);
#5508=ORIENTED_EDGE('',*,*,#4093,.T.);
#5509=ORIENTED_EDGE('',*,*,#4090,.T.);
#5510=ORIENTED_EDGE('',*,*,#4087,.T.);
#5511=ORIENTED_EDGE('',*,*,#4084,.T.);
#5512=ORIENTED_EDGE('',*,*,#4081,.T.);
#5513=ORIENTED_EDGE('',*,*,#4078,.T.);
#5514=ORIENTED_EDGE('',*,*,#4075,.T.);
#5515=ORIENTED_EDGE('',*,*,#4072,.T.);
#5516=ORIENTED_EDGE('',*,*,#4069,.T.);
#5517=ORIENTED_EDGE('',*,*,#4066,.T.);
#5518=ORIENTED_EDGE('',*,*,#4063,.T.);
#5519=ORIENTED_EDGE('',*,*,#4060,.T.);
#5520=ORIENTED_EDGE('',*,*,#4057,.T.);
#5521=ORIENTED_EDGE('',*,*,#4054,.T.);
#5522=ORIENTED_EDGE('',*,*,#4051,.T.);
#5523=ORIENTED_EDGE('',*,*,#4048,.T.);
#5524=ORIENTED_EDGE('',*,*,#4045,.T.);
#5525=ORIENTED_EDGE('',*,*,#4042,.T.);
#5526=ORIENTED_EDGE('',*,*,#4039,.T.);
#5527=ORIENTED_EDGE('',*,*,#4036,.T.);
#5528=ORIENTED_EDGE('',*,*,#4033,.T.);
#5529=ORIENTED_EDGE('',*,*,#4030,.T.);
#5530=ORIENTED_EDGE('',*,*,#4027,.T.);
#5531=ORIENTED_EDGE('',*,*,#4024,.T.);
#5532=ORIENTED_EDGE('',*,*,#4021,.T.);
#5533=ORIENTED_EDGE('',*,*,#4018,.T.);
#5534=ORIENTED_EDGE('',*,*,#4015,.T.);
#5535=ORIENTED_EDGE('',*,*,#4012,.T.);
#5536=ORIENTED_EDGE('',*,*,#4009,.T.);
#5537=ORIENTED_EDGE('',*,*,#4006,.T.);
#5538=ORIENTED_EDGE('',*,*,#4003,.T.);
#5539=ORIENTED_EDGE('',*,*,#4000,.T.);
#5540=ORIENTED_EDGE('',*,*,#3997,.T.);
#5541=ORIENTED_EDGE('',*,*,#3991,.T.);
#5542=ORIENTED_EDGE('',*,*,#4137,.T.);
#5543=ORIENTED_EDGE('',*,*,#3995,.T.);
#5544=ORIENTED_EDGE('',*,*,#3999,.T.);
#5545=ORIENTED_EDGE('',*,*,#4002,.T.);
#5546=ORIENTED_EDGE('',*,*,#4005,.T.);
#5547=ORIENTED_EDGE('',*,*,#4008,.T.);
#5548=ORIENTED_EDGE('',*,*,#4011,.T.);
#5549=ORIENTED_EDGE('',*,*,#4014,.T.);
#5550=ORIENTED_EDGE('',*,*,#4017,.T.);
#5551=ORIENTED_EDGE('',*,*,#4020,.T.);
#5552=ORIENTED_EDGE('',*,*,#4023,.T.);
#5553=ORIENTED_EDGE('',*,*,#4026,.T.);
#5554=ORIENTED_EDGE('',*,*,#4029,.T.);
#5555=ORIENTED_EDGE('',*,*,#4032,.T.);
#5556=ORIENTED_EDGE('',*,*,#4035,.T.);
#5557=ORIENTED_EDGE('',*,*,#4038,.T.);
#5558=ORIENTED_EDGE('',*,*,#4041,.T.);
#5559=ORIENTED_EDGE('',*,*,#4044,.T.);
#5560=ORIENTED_EDGE('',*,*,#4047,.T.);
#5561=ORIENTED_EDGE('',*,*,#4050,.T.);
#5562=ORIENTED_EDGE('',*,*,#4053,.T.);
#5563=ORIENTED_EDGE('',*,*,#4056,.T.);
#5564=ORIENTED_EDGE('',*,*,#4059,.T.);
#5565=ORIENTED_EDGE('',*,*,#4062,.T.);
#5566=ORIENTED_EDGE('',*,*,#4065,.T.);
#5567=ORIENTED_EDGE('',*,*,#4068,.T.);
#5568=ORIENTED_EDGE('',*,*,#4071,.T.);
#5569=ORIENTED_EDGE('',*,*,#4074,.T.);
#5570=ORIENTED_EDGE('',*,*,#4077,.T.);
#5571=ORIENTED_EDGE('',*,*,#4080,.T.);
#5572=ORIENTED_EDGE('',*,*,#4083,.T.);
#5573=ORIENTED_EDGE('',*,*,#4086,.T.);
#5574=ORIENTED_EDGE('',*,*,#4089,.T.);
#5575=ORIENTED_EDGE('',*,*,#4092,.T.);
#5576=ORIENTED_EDGE('',*,*,#4095,.T.);
#5577=ORIENTED_EDGE('',*,*,#4098,.T.);
#5578=ORIENTED_EDGE('',*,*,#4101,.T.);
#5579=ORIENTED_EDGE('',*,*,#4104,.T.);
#5580=ORIENTED_EDGE('',*,*,#4107,.T.);
#5581=ORIENTED_EDGE('',*,*,#4110,.T.);
#5582=ORIENTED_EDGE('',*,*,#4113,.T.);
#5583=ORIENTED_EDGE('',*,*,#4116,.T.);
#5584=ORIENTED_EDGE('',*,*,#4119,.T.);
#5585=ORIENTED_EDGE('',*,*,#4122,.T.);
#5586=ORIENTED_EDGE('',*,*,#4125,.T.);
#5587=ORIENTED_EDGE('',*,*,#4128,.T.);
#5588=ORIENTED_EDGE('',*,*,#4131,.T.);
#5589=ORIENTED_EDGE('',*,*,#4134,.T.);
#5590=ORIENTED_EDGE('',*,*,#3993,.T.);
#5896=CYLINDRICAL_SURFACE('',#7146,0.21);
#5897=CYLINDRICAL_SURFACE('',#7150,1.6);
#5898=CYLINDRICAL_SURFACE('',#7155,1.005);
#6156=ADVANCED_FACE('',(#1086),#750,.T.);
#6157=ADVANCED_FACE('',(#1087),#5896,.F.);
#6158=ADVANCED_FACE('',(#1088),#751,.T.);
#6159=ADVANCED_FACE('',(#1089,#586),#5897,.T.);
#6160=ADVANCED_FACE('',(#1090,#587),#752,.T.);
#6161=ADVANCED_FACE('',(#1091,#588),#5898,.F.);
#6162=ADVANCED_FACE('',(#1092),#753,.T.);
#6163=ADVANCED_FACE('',(#1093),#754,.T.);
#6164=ADVANCED_FACE('',(#1094),#755,.T.);
#6165=ADVANCED_FACE('',(#1095),#756,.T.);
#6166=ADVANCED_FACE('',(#1096),#757,.T.);
#6167=ADVANCED_FACE('',(#1097),#758,.T.);
#6168=ADVANCED_FACE('',(#1098),#759,.T.);
#6169=ADVANCED_FACE('',(#1099),#760,.T.);
#6170=ADVANCED_FACE('',(#1100),#761,.T.);
#6171=ADVANCED_FACE('',(#1101),#762,.T.);
#6172=ADVANCED_FACE('',(#1102),#763,.T.);
#6173=ADVANCED_FACE('',(#1103),#764,.T.);
#6174=ADVANCED_FACE('',(#1104),#765,.T.);
#6175=ADVANCED_FACE('',(#1105),#766,.T.);
#6176=ADVANCED_FACE('',(#1106),#767,.T.);
#6177=ADVANCED_FACE('',(#1107),#768,.T.);
#6178=ADVANCED_FACE('',(#1108),#769,.T.);
#6179=ADVANCED_FACE('',(#1109),#770,.T.);
#6180=ADVANCED_FACE('',(#1110),#771,.T.);
#6181=ADVANCED_FACE('',(#1111),#772,.T.);
#6182=ADVANCED_FACE('',(#1112),#773,.T.);
#6183=ADVANCED_FACE('',(#1113),#774,.T.);
#6184=ADVANCED_FACE('',(#1114),#775,.T.);
#6185=ADVANCED_FACE('',(#1115),#776,.T.);
#6186=ADVANCED_FACE('',(#1116),#777,.T.);
#6187=ADVANCED_FACE('',(#1117),#778,.T.);
#6188=ADVANCED_FACE('',(#1118),#779,.T.);
#6189=ADVANCED_FACE('',(#1119),#780,.T.);
#6190=ADVANCED_FACE('',(#1120),#781,.T.);
#6191=ADVANCED_FACE('',(#1121),#782,.T.);
#6192=ADVANCED_FACE('',(#1122),#783,.T.);
#6193=ADVANCED_FACE('',(#1123),#784,.T.);
#6194=ADVANCED_FACE('',(#1124),#785,.T.);
#6195=ADVANCED_FACE('',(#1125),#786,.T.);
#6196=ADVANCED_FACE('',(#1126),#787,.T.);
#6197=ADVANCED_FACE('',(#1127),#788,.T.);
#6198=ADVANCED_FACE('',(#1128),#789,.T.);
#6199=ADVANCED_FACE('',(#1129),#790,.T.);
#6200=ADVANCED_FACE('',(#1130),#791,.T.);
#6201=ADVANCED_FACE('',(#1131),#792,.T.);
#6202=ADVANCED_FACE('',(#1132),#793,.T.);
#6203=ADVANCED_FACE('',(#1133),#794,.T.);
#6204=ADVANCED_FACE('',(#1134),#795,.T.);
#6205=ADVANCED_FACE('',(#1135),#796,.T.);
#6206=ADVANCED_FACE('',(#1136),#797,.T.);
#6207=ADVANCED_FACE('',(#1137),#798,.T.);
#6208=ADVANCED_FACE('',(#1138),#799,.T.);
#6209=ADVANCED_FACE('',(#1139),#800,.T.);
#6210=ADVANCED_FACE('',(#1140,#589),#801,.T.);
#6211=ADVANCED_FACE('',(#1141,#590),#802,.F.);
#6297=CLOSED_SHELL('',(#6156,#6157,#6158,#6159,#6160,#6161,#6162,#6163,
#6164,#6165,#6166,#6167,#6168,#6169,#6170,#6171,#6172,#6173,#6174,#6175,
#6176,#6177,#6178,#6179,#6180,#6181,#6182,#6183,#6184,#6185,#6186,#6187,
#6188,#6189,#6190,#6191,#6192,#6193,#6194,#6195,#6196,#6197,#6198,#6199,
#6200,#6201,#6202,#6203,#6204,#6205,#6206,#6207,#6208,#6209,#6210,#6211));
#7143=AXIS2_PLACEMENT_3D('',#11015,#8574,#8575);
#7144=AXIS2_PLACEMENT_3D('',#11016,#8576,#8577);
#7145=AXIS2_PLACEMENT_3D('',#11020,#8579,#8580);
#7146=AXIS2_PLACEMENT_3D('',#11021,#8581,#8582);
#7147=AXIS2_PLACEMENT_3D('',#11038,#8583,#8584);
#7148=AXIS2_PLACEMENT_3D('',#11079,#8586,#8587);
#7149=AXIS2_PLACEMENT_3D('',#11094,#8588,#8589);
#7150=AXIS2_PLACEMENT_3D('',#11096,#8591,#8592);
#7151=AXIS2_PLACEMENT_3D('',#11098,#8593,#8594);
#7152=AXIS2_PLACEMENT_3D('',#11101,#8596,#8597);
#7153=AXIS2_PLACEMENT_3D('',#11102,#8598,#8599);
#7154=AXIS2_PLACEMENT_3D('',#11104,#8600,#8601);
#7155=AXIS2_PLACEMENT_3D('',#11105,#8602,#8603);
#7156=AXIS2_PLACEMENT_3D('',#11107,#8604,#8605);
#7157=AXIS2_PLACEMENT_3D('',#11109,#8607,#8608);
#7158=AXIS2_PLACEMENT_3D('',#11118,#8613,#8614);
#7159=AXIS2_PLACEMENT_3D('',#11124,#8618,#8619);
#7160=AXIS2_PLACEMENT_3D('',#11130,#8623,#8624);
#7161=AXIS2_PLACEMENT_3D('',#11136,#8628,#8629);
#7162=AXIS2_PLACEMENT_3D('',#11142,#8633,#8634);
#7163=AXIS2_PLACEMENT_3D('',#11148,#8638,#8639);
#7164=AXIS2_PLACEMENT_3D('',#11154,#8643,#8644);
#7165=AXIS2_PLACEMENT_3D('',#11160,#8648,#8649);
#7166=AXIS2_PLACEMENT_3D('',#11166,#8653,#8654);
#7167=AXIS2_PLACEMENT_3D('',#11172,#8658,#8659);
#7168=AXIS2_PLACEMENT_3D('',#11178,#8663,#8664);
#7169=AXIS2_PLACEMENT_3D('',#11184,#8668,#8669);
#7170=AXIS2_PLACEMENT_3D('',#11190,#8673,#8674);
#7171=AXIS2_PLACEMENT_3D('',#11196,#8678,#8679);
#7172=AXIS2_PLACEMENT_3D('',#11202,#8683,#8684);
#7173=AXIS2_PLACEMENT_3D('',#11208,#8688,#8689);
#7174=AXIS2_PLACEMENT_3D('',#11214,#8693,#8694);
#7175=AXIS2_PLACEMENT_3D('',#11220,#8698,#8699);
#7176=AXIS2_PLACEMENT_3D('',#11226,#8703,#8704);
#7177=AXIS2_PLACEMENT_3D('',#11232,#8708,#8709);
#7178=AXIS2_PLACEMENT_3D('',#11238,#8713,#8714);
#7179=AXIS2_PLACEMENT_3D('',#11244,#8718,#8719);
#7180=AXIS2_PLACEMENT_3D('',#11250,#8723,#8724);
#7181=AXIS2_PLACEMENT_3D('',#11256,#8728,#8729);
#7182=AXIS2_PLACEMENT_3D('',#11262,#8733,#8734);
#7183=AXIS2_PLACEMENT_3D('',#11268,#8738,#8739);
#7184=AXIS2_PLACEMENT_3D('',#11274,#8743,#8744);
#7185=AXIS2_PLACEMENT_3D('',#11280,#8748,#8749);
#7186=AXIS2_PLACEMENT_3D('',#11286,#8753,#8754);
#7187=AXIS2_PLACEMENT_3D('',#11292,#8758,#8759);
#7188=AXIS2_PLACEMENT_3D('',#11298,#8763,#8764);
#7189=AXIS2_PLACEMENT_3D('',#11304,#8768,#8769);
#7190=AXIS2_PLACEMENT_3D('',#11310,#8773,#8774);
#7191=AXIS2_PLACEMENT_3D('',#11316,#8778,#8779);
#7192=AXIS2_PLACEMENT_3D('',#11322,#8783,#8784);
#7193=AXIS2_PLACEMENT_3D('',#11328,#8788,#8789);
#7194=AXIS2_PLACEMENT_3D('',#11334,#8793,#8794);
#7195=AXIS2_PLACEMENT_3D('',#11340,#8798,#8799);
#7196=AXIS2_PLACEMENT_3D('',#11346,#8803,#8804);
#7197=AXIS2_PLACEMENT_3D('',#11352,#8808,#8809);
#7198=AXIS2_PLACEMENT_3D('',#11358,#8813,#8814);
#7199=AXIS2_PLACEMENT_3D('',#11364,#8818,#8819);
#7200=AXIS2_PLACEMENT_3D('',#11370,#8823,#8824);
#7201=AXIS2_PLACEMENT_3D('',#11376,#8828,#8829);
#7202=AXIS2_PLACEMENT_3D('',#11382,#8833,#8834);
#7203=AXIS2_PLACEMENT_3D('',#11388,#8838,#8839);
#7204=AXIS2_PLACEMENT_3D('',#11394,#8843,#8844);
#7205=AXIS2_PLACEMENT_3D('',#11397,#8847,#8848);
#7206=AXIS2_PLACEMENT_3D('',#11398,#8849,#8850);
#8574=DIRECTION('axis',(0.,0.,1.));
#8575=DIRECTION('refdir',(1.,0.,0.));
#8576=DIRECTION('center_axis',(0.,0.,1.));
#8577=DIRECTION('ref_axis',(1.,0.,0.));
#8578=DIRECTION('',(0.,1.,0.));
#8579=DIRECTION('center_axis',(0.,0.,1.));
#8580=DIRECTION('ref_axis',(1.,0.,0.));
#8581=DIRECTION('center_axis',(0.,0.,1.));
#8582=DIRECTION('ref_axis',(1.,0.,0.));
#8583=DIRECTION('center_axis',(0.,0.,1.));
#8584=DIRECTION('ref_axis',(1.,0.,0.));
#8585=DIRECTION('',(0.,0.,1.));
#8586=DIRECTION('center_axis',(0.,0.,1.));
#8587=DIRECTION('ref_axis',(1.,0.,0.));
#8588=DIRECTION('center_axis',(0.,0.,1.));
#8589=DIRECTION('ref_axis',(1.,0.,0.));
#8590=DIRECTION('',(0.,-1.,0.));
#8591=DIRECTION('center_axis',(0.,1.,0.));
#8592=DIRECTION('ref_axis',(1.,0.,0.));
#8593=DIRECTION('center_axis',(0.,1.,0.));
#8594=DIRECTION('ref_axis',(1.,0.,0.));
#8595=DIRECTION('',(0.,-1.,0.));
#8596=DIRECTION('center_axis',(0.,-1.,0.));
#8597=DIRECTION('ref_axis',(1.,0.,0.));
#8598=DIRECTION('center_axis',(0.,1.,0.));
#8599=DIRECTION('ref_axis',(1.,0.,0.));
#8600=DIRECTION('center_axis',(0.,-1.,0.));
#8601=DIRECTION('ref_axis',(1.,0.,0.));
#8602=DIRECTION('center_axis',(0.,1.,0.));
#8603=DIRECTION('ref_axis',(1.,0.,0.));
#8604=DIRECTION('center_axis',(0.,1.,0.));
#8605=DIRECTION('ref_axis',(1.,0.,0.));
#8606=DIRECTION('',(0.,1.,0.));
#8607=DIRECTION('center_axis',(0.015706233006771,0.,0.999876649514697));
#8608=DIRECTION('ref_axis',(0.999876649514697,0.,-0.015706233006771));
#8609=DIRECTION('',(-0.999876649514697,0.,0.015706233006771));
#8610=DIRECTION('',(0.,1.,0.));
#8611=DIRECTION('',(0.999876649514697,0.,-0.015706233006771));
#8612=DIRECTION('',(0.,1.,0.));
#8613=DIRECTION('center_axis',(0.957469564385932,0.,-0.288534284400681));
#8614=DIRECTION('ref_axis',(-0.288534284400681,0.,-0.957469564385932));
#8615=DIRECTION('',(0.288534284400681,0.,0.957469564385932));
#8616=DIRECTION('',(-0.288534284400681,0.,-0.957469564385932));
#8617=DIRECTION('',(0.,1.,0.));
#8618=DIRECTION('center_axis',(-0.243616063552747,0.,0.9698717510986));
#8619=DIRECTION('ref_axis',(0.9698717510986,0.,0.243616063552747));
#8620=DIRECTION('',(-0.9698717510986,0.,-0.243616063552747));
#8621=DIRECTION('',(0.9698717510986,0.,0.243616063552747));
#8622=DIRECTION('',(0.,1.,0.));
#8623=DIRECTION('center_axis',(0.999522748094039,0.,-0.0308913587033594));
#8624=DIRECTION('ref_axis',(-0.0308913587033594,0.,-0.999522748094039));
#8625=DIRECTION('',(0.0308913587033594,0.,0.999522748094039));
#8626=DIRECTION('',(-0.0308913587033594,0.,-0.999522748094039));
#8627=DIRECTION('',(0.,1.,0.));
#8628=DIRECTION('center_axis',(-0.486336327975727,0.,0.873771695633983));
#8629=DIRECTION('ref_axis',(0.873771695633983,0.,0.486336327975727));
#8630=DIRECTION('',(-0.873771695633983,0.,-0.486336327975727));
#8631=DIRECTION('',(0.873771695633983,0.,0.486336327975727));
#8632=DIRECTION('',(0.,1.,0.));
#8633=DIRECTION('center_axis',(0.973460108308978,0.,0.228856762039213));
#8634=DIRECTION('ref_axis',(0.228856762039213,0.,-0.973460108308978));
#8635=DIRECTION('',(-0.228856762039213,0.,0.973460108308978));
#8636=DIRECTION('',(0.228856762039213,0.,-0.973460108308978));
#8637=DIRECTION('',(0.,1.,0.));
#8638=DIRECTION('center_axis',(-0.695913575355945,0.,0.71812554308791));
#8639=DIRECTION('ref_axis',(0.71812554308791,0.,0.695913575355945));
#8640=DIRECTION('',(-0.71812554308791,0.,-0.695913575355945));
#8641=DIRECTION('',(0.71812554308791,0.,0.695913575355945));
#8642=DIRECTION('',(0.,1.,0.));
#8643=DIRECTION('center_axis',(0.881057770861552,0.,0.473008672652493));
#8644=DIRECTION('ref_axis',(0.473008672652493,0.,-0.881057770861552));
#8645=DIRECTION('',(-0.473008672652493,0.,0.881057770861552));
#8646=DIRECTION('',(0.473008672652493,0.,-0.881057770861552));
#8647=DIRECTION('',(0.,1.,0.));
#8648=DIRECTION('center_axis',(-0.858065462627213,0.,0.513540321538968));
#8649=DIRECTION('ref_axis',(0.513540321538968,0.,0.858065462627213));
#8650=DIRECTION('',(-0.513540321538968,0.,-0.858065462627213));
#8651=DIRECTION('',(0.513540321538968,0.,0.858065462627213));
#8652=DIRECTION('',(0.,1.,0.));
#8653=DIRECTION('center_axis',(0.728612802346719,0.,0.684925823908298));
#8654=DIRECTION('ref_axis',(0.684925823908298,0.,-0.728612802346719));
#8655=DIRECTION('',(-0.684925823908298,0.,0.728612802346719));
#8656=DIRECTION('',(0.684925823908298,0.,-0.728612802346719));
#8657=DIRECTION('',(0.,1.,0.));
#8658=DIRECTION('center_axis',(-0.96174160664066,0.,0.273958175742654));
#8659=DIRECTION('ref_axis',(0.273958175742654,0.,0.96174160664066));
#8660=DIRECTION('',(-0.273958175742654,0.,-0.96174160664066));
#8661=DIRECTION('',(0.273958175742654,0.,0.96174160664066));
#8662=DIRECTION('',(0.,1.,0.));
#8663=DIRECTION('center_axis',(0.526514075441545,0.,0.850166412158193));
#8664=DIRECTION('ref_axis',(0.850166412158193,0.,-0.526514075441545));
#8665=DIRECTION('',(-0.850166412158193,0.,0.526514075441545));
#8666=DIRECTION('',(0.850166412158193,0.,-0.526514075441545));
#8667=DIRECTION('',(0.,1.,0.));
#8668=DIRECTION('center_axis',(-0.999876649514698,0.,0.0157062330067685));
#8669=DIRECTION('ref_axis',(0.0157062330067685,0.,0.999876649514698));
#8670=DIRECTION('',(-0.0157062330067685,0.,-0.999876649514698));
#8671=DIRECTION('',(0.0157062330067685,0.,0.999876649514698));
#8672=DIRECTION('',(0.,1.,0.));
#8673=DIRECTION('center_axis',(0.288534284400681,0.,0.957469564385932));
#8674=DIRECTION('ref_axis',(0.957469564385932,0.,-0.288534284400681));
#8675=DIRECTION('',(-0.957469564385932,0.,0.288534284400681));
#8676=DIRECTION('',(0.957469564385932,0.,-0.288534284400681));
#8677=DIRECTION('',(0.,1.,0.));
#8678=DIRECTION('center_axis',(-0.969871751098599,0.,-0.243616063552749));
#8679=DIRECTION('ref_axis',(-0.243616063552749,0.,0.969871751098599));
#8680=DIRECTION('',(0.243616063552749,0.,-0.969871751098599));
#8681=DIRECTION('',(-0.243616063552749,0.,0.969871751098599));
#8682=DIRECTION('',(0.,1.,0.));
#8683=DIRECTION('center_axis',(0.0308913587033598,0.,0.999522748094039));
#8684=DIRECTION('ref_axis',(0.999522748094039,0.,-0.0308913587033598));
#8685=DIRECTION('',(-0.999522748094039,0.,0.0308913587033598));
#8686=DIRECTION('',(0.999522748094039,0.,-0.0308913587033598));
#8687=DIRECTION('',(0.,1.,0.));
#8688=DIRECTION('center_axis',(-0.873771695633983,0.,-0.486336327975728));
#8689=DIRECTION('ref_axis',(-0.486336327975728,0.,0.873771695633983));
#8690=DIRECTION('',(0.486336327975728,0.,-0.873771695633983));
#8691=DIRECTION('',(-0.486336327975728,0.,0.873771695633983));
#8692=DIRECTION('',(0.,1.,0.));
#8693=DIRECTION('center_axis',(-0.228856762039212,0.,0.973460108308978));
#8694=DIRECTION('ref_axis',(0.973460108308978,0.,0.228856762039212));
#8695=DIRECTION('',(-0.973460108308978,0.,-0.228856762039212));
#8696=DIRECTION('',(0.973460108308978,0.,0.228856762039212));
#8697=DIRECTION('',(0.,1.,0.));
#8698=DIRECTION('center_axis',(-0.718125543087911,0.,-0.695913575355944));
#8699=DIRECTION('ref_axis',(-0.695913575355944,0.,0.718125543087911));
#8700=DIRECTION('',(0.695913575355944,0.,-0.718125543087911));
#8701=DIRECTION('',(-0.695913575355944,0.,0.718125543087911));
#8702=DIRECTION('',(0.,1.,0.));
#8703=DIRECTION('center_axis',(-0.473008672652494,0.,0.881057770861551));
#8704=DIRECTION('ref_axis',(0.881057770861551,0.,0.473008672652494));
#8705=DIRECTION('',(-0.881057770861551,0.,-0.473008672652494));
#8706=DIRECTION('',(0.881057770861551,0.,0.473008672652494));
#8707=DIRECTION('',(0.,1.,0.));
#8708=DIRECTION('center_axis',(-0.513540321538967,0.,-0.858065462627214));
#8709=DIRECTION('ref_axis',(-0.858065462627214,0.,0.513540321538967));
#8710=DIRECTION('',(0.858065462627214,0.,-0.513540321538967));
#8711=DIRECTION('',(-0.858065462627214,0.,0.513540321538967));
#8712=DIRECTION('',(0.,1.,0.));
#8713=DIRECTION('center_axis',(-0.684925823908296,0.,0.728612802346721));
#8714=DIRECTION('ref_axis',(0.728612802346721,0.,0.684925823908296));
#8715=DIRECTION('',(-0.728612802346721,0.,-0.684925823908296));
#8716=DIRECTION('',(0.728612802346721,0.,0.684925823908296));
#8717=DIRECTION('',(0.,1.,0.));
#8718=DIRECTION('center_axis',(-0.273958175742656,0.,-0.961741606640659));
#8719=DIRECTION('ref_axis',(-0.961741606640659,0.,0.273958175742656));
#8720=DIRECTION('',(0.961741606640659,0.,-0.273958175742656));
#8721=DIRECTION('',(-0.961741606640659,0.,0.273958175742656));
#8722=DIRECTION('',(0.,1.,0.));
#8723=DIRECTION('center_axis',(-0.850166412158193,0.,0.526514075441546));
#8724=DIRECTION('ref_axis',(0.526514075441546,0.,0.850166412158193));
#8725=DIRECTION('',(-0.526514075441546,0.,-0.850166412158193));
#8726=DIRECTION('',(0.526514075441546,0.,0.850166412158193));
#8727=DIRECTION('',(0.,1.,0.));
#8728=DIRECTION('center_axis',(-0.0157062330067692,0.,-0.999876649514697));
#8729=DIRECTION('ref_axis',(-0.999876649514697,0.,0.0157062330067692));
#8730=DIRECTION('',(0.999876649514697,0.,-0.0157062330067692));
#8731=DIRECTION('',(-0.999876649514697,0.,0.0157062330067692));
#8732=DIRECTION('',(0.,1.,0.));
#8733=DIRECTION('center_axis',(-0.957469564385932,0.,0.288534284400681));
#8734=DIRECTION('ref_axis',(0.288534284400681,0.,0.957469564385932));
#8735=DIRECTION('',(-0.288534284400681,0.,-0.957469564385932));
#8736=DIRECTION('',(0.288534284400681,0.,0.957469564385932));
#8737=DIRECTION('',(0.,1.,0.));
#8738=DIRECTION('center_axis',(0.24361606355275,0.,-0.969871751098599));
#8739=DIRECTION('ref_axis',(-0.969871751098599,0.,-0.24361606355275));
#8740=DIRECTION('',(0.969871751098599,0.,0.24361606355275));
#8741=DIRECTION('',(-0.969871751098599,0.,-0.24361606355275));
#8742=DIRECTION('',(0.,1.,0.));
#8743=DIRECTION('center_axis',(-0.999522748094039,0.,0.0308913587033594));
#8744=DIRECTION('ref_axis',(0.0308913587033594,0.,0.999522748094039));
#8745=DIRECTION('',(-0.0308913587033594,0.,-0.999522748094039));
#8746=DIRECTION('',(0.0308913587033594,0.,0.999522748094039));
#8747=DIRECTION('',(0.,1.,0.));
#8748=DIRECTION('center_axis',(0.486336327975727,0.,-0.873771695633983));
#8749=DIRECTION('ref_axis',(-0.873771695633983,0.,-0.486336327975727));
#8750=DIRECTION('',(0.873771695633983,0.,0.486336327975727));
#8751=DIRECTION('',(-0.873771695633983,0.,-0.486336327975727));
#8752=DIRECTION('',(0.,1.,0.));
#8753=DIRECTION('center_axis',(-0.973460108308978,0.,-0.228856762039212));
#8754=DIRECTION('ref_axis',(-0.228856762039212,0.,0.973460108308978));
#8755=DIRECTION('',(0.228856762039212,0.,-0.973460108308978));
#8756=DIRECTION('',(-0.228856762039212,0.,0.973460108308978));
#8757=DIRECTION('',(0.,1.,0.));
#8758=DIRECTION('center_axis',(0.695913575355945,0.,-0.718125543087909));
#8759=DIRECTION('ref_axis',(-0.718125543087909,0.,-0.695913575355945));
#8760=DIRECTION('',(0.718125543087909,0.,0.695913575355945));
#8761=DIRECTION('',(-0.718125543087909,0.,-0.695913575355945));
#8762=DIRECTION('',(0.,1.,0.));
#8763=DIRECTION('center_axis',(-0.881057770861552,0.,-0.473008672652493));
#8764=DIRECTION('ref_axis',(-0.473008672652493,0.,0.881057770861552));
#8765=DIRECTION('',(0.473008672652493,0.,-0.881057770861552));
#8766=DIRECTION('',(-0.473008672652493,0.,0.881057770861552));
#8767=DIRECTION('',(0.,1.,0.));
#8768=DIRECTION('center_axis',(0.858065462627214,0.,-0.513540321538968));
#8769=DIRECTION('ref_axis',(-0.513540321538968,0.,-0.858065462627214));
#8770=DIRECTION('',(0.513540321538968,0.,0.858065462627214));
#8771=DIRECTION('',(-0.513540321538968,0.,-0.858065462627214));
#8772=DIRECTION('',(0.,1.,0.));
#8773=DIRECTION('center_axis',(-0.728612802346719,0.,-0.684925823908298));
#8774=DIRECTION('ref_axis',(-0.684925823908298,0.,0.728612802346719));
#8775=DIRECTION('',(0.684925823908298,0.,-0.728612802346719));
#8776=DIRECTION('',(-0.684925823908298,0.,0.728612802346719));
#8777=DIRECTION('',(0.,1.,0.));
#8778=DIRECTION('center_axis',(0.96174160664066,0.,-0.273958175742653));
#8779=DIRECTION('ref_axis',(-0.273958175742653,0.,-0.96174160664066));
#8780=DIRECTION('',(0.273958175742653,0.,0.96174160664066));
#8781=DIRECTION('',(-0.273958175742653,0.,-0.96174160664066));
#8782=DIRECTION('',(0.,1.,0.));
#8783=DIRECTION('center_axis',(-0.526514075441546,0.,-0.850166412158193));
#8784=DIRECTION('ref_axis',(-0.850166412158193,0.,0.526514075441546));
#8785=DIRECTION('',(0.850166412158193,0.,-0.526514075441546));
#8786=DIRECTION('',(-0.850166412158193,0.,0.526514075441546));
#8787=DIRECTION('',(0.,1.,0.));
#8788=DIRECTION('center_axis',(0.999876649514698,0.,-0.0157062330067686));
#8789=DIRECTION('ref_axis',(-0.0157062330067686,0.,-0.999876649514698));
#8790=DIRECTION('',(0.0157062330067686,0.,0.999876649514698));
#8791=DIRECTION('',(-0.0157062330067686,0.,-0.999876649514698));
#8792=DIRECTION('',(0.,1.,0.));
#8793=DIRECTION('center_axis',(-0.288534284400682,0.,-0.957469564385932));
#8794=DIRECTION('ref_axis',(-0.957469564385932,0.,0.288534284400682));
#8795=DIRECTION('',(0.957469564385932,0.,-0.288534284400682));
#8796=DIRECTION('',(-0.957469564385932,0.,0.288534284400682));
#8797=DIRECTION('',(0.,1.,0.));
#8798=DIRECTION('center_axis',(0.969871751098599,0.,0.24361606355275));
#8799=DIRECTION('ref_axis',(0.24361606355275,0.,-0.969871751098599));
#8800=DIRECTION('',(-0.24361606355275,0.,0.969871751098599));
#8801=DIRECTION('',(0.24361606355275,0.,-0.969871751098599));
#8802=DIRECTION('',(0.,1.,0.));
#8803=DIRECTION('center_axis',(-0.0308913587033594,0.,-0.999522748094039));
#8804=DIRECTION('ref_axis',(-0.999522748094039,0.,0.0308913587033594));
#8805=DIRECTION('',(0.999522748094039,0.,-0.0308913587033594));
#8806=DIRECTION('',(-0.999522748094039,0.,0.0308913587033594));
#8807=DIRECTION('',(0.,1.,0.));
#8808=DIRECTION('center_axis',(0.873771695633986,0.,0.486336327975723));
#8809=DIRECTION('ref_axis',(0.486336327975723,0.,-0.873771695633986));
#8810=DIRECTION('',(-0.486336327975723,0.,0.873771695633986));
#8811=DIRECTION('',(0.486336327975723,0.,-0.873771695633986));
#8812=DIRECTION('',(0.,1.,0.));
#8813=DIRECTION('center_axis',(0.228856762039213,0.,-0.973460108308978));
#8814=DIRECTION('ref_axis',(-0.973460108308978,0.,-0.228856762039213));
#8815=DIRECTION('',(0.973460108308978,0.,0.228856762039213));
#8816=DIRECTION('',(-0.973460108308978,0.,-0.228856762039213));
#8817=DIRECTION('',(0.,1.,0.));
#8818=DIRECTION('center_axis',(0.718125543087909,0.,0.695913575355946));
#8819=DIRECTION('ref_axis',(0.695913575355946,0.,-0.718125543087909));
#8820=DIRECTION('',(-0.695913575355946,0.,0.718125543087909));
#8821=DIRECTION('',(0.695913575355946,0.,-0.718125543087909));
#8822=DIRECTION('',(0.,1.,0.));
#8823=DIRECTION('center_axis',(0.473008672652493,0.,-0.881057770861552));
#8824=DIRECTION('ref_axis',(-0.881057770861552,0.,-0.473008672652493));
#8825=DIRECTION('',(0.881057770861552,0.,0.473008672652493));
#8826=DIRECTION('',(-0.881057770861552,0.,-0.473008672652493));
#8827=DIRECTION('',(0.,1.,0.));
#8828=DIRECTION('center_axis',(0.513540321538969,0.,0.858065462627213));
#8829=DIRECTION('ref_axis',(0.858065462627213,0.,-0.513540321538969));
#8830=DIRECTION('',(-0.858065462627213,0.,0.513540321538969));
#8831=DIRECTION('',(0.858065462627213,0.,-0.513540321538969));
#8832=DIRECTION('',(0.,1.,0.));
#8833=DIRECTION('center_axis',(0.684925823908296,0.,-0.728612802346721));
#8834=DIRECTION('ref_axis',(-0.728612802346721,0.,-0.684925823908296));
#8835=DIRECTION('',(0.728612802346721,0.,0.684925823908296));
#8836=DIRECTION('',(-0.728612802346721,0.,-0.684925823908296));
#8837=DIRECTION('',(0.,1.,0.));
#8838=DIRECTION('center_axis',(0.27395817574266,0.,0.961741606640658));
#8839=DIRECTION('ref_axis',(0.961741606640658,0.,-0.27395817574266));
#8840=DIRECTION('',(-0.961741606640658,0.,0.27395817574266));
#8841=DIRECTION('',(0.961741606640658,0.,-0.27395817574266));
#8842=DIRECTION('',(0.,1.,0.));
#8843=DIRECTION('center_axis',(0.850166412158193,0.,-0.526514075441546));
#8844=DIRECTION('ref_axis',(-0.526514075441546,0.,-0.850166412158193));
#8845=DIRECTION('',(0.526514075441546,0.,0.850166412158193));
#8846=DIRECTION('',(-0.526514075441546,0.,-0.850166412158193));
#8847=DIRECTION('center_axis',(0.,1.,0.));
#8848=DIRECTION('ref_axis',(0.,0.,1.));
#8849=DIRECTION('center_axis',(0.,1.,0.));
#8850=DIRECTION('ref_axis',(1.,0.,0.));
#11015=CARTESIAN_POINT('',(0.,0.,0.));
#11016=CARTESIAN_POINT('Origin',(0.,-2.4,7.52));
#11017=CARTESIAN_POINT('',(0.172988438920056,-2.51905880899792,7.52));
#11018=CARTESIAN_POINT('',(0.172988438920056,-2.28094119100208,7.52));
#11019=CARTESIAN_POINT('',(0.172988438920056,-3.6,7.52));
#11020=CARTESIAN_POINT('Origin',(0.,-2.4,7.52));
#11021=CARTESIAN_POINT('Origin',(0.,-2.4,7.52));
#11022=CARTESIAN_POINT('',(-0.172988438920056,-2.51905880899792,7.52));
#11023=CARTESIAN_POINT('Ctrl Pts',(-0.172988438920056,-2.51905880899792,
7.52));
#11024=CARTESIAN_POINT('Ctrl Pts',(-0.165594865311314,-2.52980142239529,
7.52129192197638));
#11025=CARTESIAN_POINT('Ctrl Pts',(-0.157297138725606,-2.53968770937274,
7.52265394943905));
#11026=CARTESIAN_POINT('Ctrl Pts',(-0.129892073845076,-2.56709277425327,
7.5267480843909));
#11027=CARTESIAN_POINT('Ctrl Pts',(-0.106330167759285,-2.58324205633295,
7.52969589327638));
#11028=CARTESIAN_POINT('Ctrl Pts',(-0.0546129046324105,-2.60469779396491,
7.53385029472357));
#11029=CARTESIAN_POINT('Ctrl Pts',(-0.0264512308298517,-2.61,7.535));
#11030=CARTESIAN_POINT('Ctrl Pts',(0.0264512308298516,-2.61,7.535));
#11031=CARTESIAN_POINT('Ctrl Pts',(0.0546129046324104,-2.60469779396491,
7.53385029472357));
#11032=CARTESIAN_POINT('Ctrl Pts',(0.106330167759284,-2.58324205633295,
7.52969589327638));
#11033=CARTESIAN_POINT('Ctrl Pts',(0.129892073845076,-2.56709277425327,
7.5267480843909));
#11034=CARTESIAN_POINT('Ctrl Pts',(0.157297138725606,-2.53968770937274,
7.52265394943905));
#11035=CARTESIAN_POINT('Ctrl Pts',(0.165594865311314,-2.52980142239529,
7.52129192197638));
#11036=CARTESIAN_POINT('Ctrl Pts',(0.172988438920056,-2.51905880899792,
7.52));
#11037=CARTESIAN_POINT('',(-0.21,-2.4,7.52));
#11038=CARTESIAN_POINT('Origin',(0.,-2.4,7.52));
#11039=CARTESIAN_POINT('',(-0.21,-2.4,8.11615888233178));
#11040=CARTESIAN_POINT('',(-0.21,-2.4,7.52));
#11041=CARTESIAN_POINT('',(0.21,-2.4,8.11615888233178));
#11042=CARTESIAN_POINT('Ctrl Pts',(0.21,-2.4,8.11615888233178));
#11043=CARTESIAN_POINT('Ctrl Pts',(0.21,-2.42640093420375,8.11615888233178));
#11044=CARTESIAN_POINT('Ctrl Pts',(0.20471752266132,-2.45454055536511,8.11688606295397));
#11045=CARTESIAN_POINT('Ctrl Pts',(0.183276841782292,-2.5062710523005,8.11950502964782));
#11046=CARTESIAN_POINT('Ctrl Pts',(0.167120287247804,-2.52986456085055,
8.12135816887013));
#11047=CARTESIAN_POINT('Ctrl Pts',(0.129864750292352,-2.567120097806,8.12483075953278));
#11048=CARTESIAN_POINT('Ctrl Pts',(0.106271159541076,-2.58327680083123,
8.12667690933009));
#11049=CARTESIAN_POINT('Ctrl Pts',(0.0545403836274688,-2.6047175903444,
8.12927985626981));
#11050=CARTESIAN_POINT('Ctrl Pts',(0.0264006657112965,-2.61,8.13));
#11051=CARTESIAN_POINT('Ctrl Pts',(-0.0264006657112964,-2.61,8.13));
#11052=CARTESIAN_POINT('Ctrl Pts',(-0.0545403836274688,-2.6047175903444,
8.12927985626981));
#11053=CARTESIAN_POINT('Ctrl Pts',(-0.106271159541076,-2.58327680083123,
8.12667690933009));
#11054=CARTESIAN_POINT('Ctrl Pts',(-0.129864750292352,-2.567120097806,8.12483075953278));
#11055=CARTESIAN_POINT('Ctrl Pts',(-0.167120287247804,-2.52986456085055,
8.12135816887013));
#11056=CARTESIAN_POINT('Ctrl Pts',(-0.183276841782292,-2.5062710523005,
8.11950502964782));
#11057=CARTESIAN_POINT('Ctrl Pts',(-0.20471752266132,-2.45454055536511,
8.11688606295397));
#11058=CARTESIAN_POINT('Ctrl Pts',(-0.21,-2.42640093420375,8.11615888233178));
#11059=CARTESIAN_POINT('Ctrl Pts',(-0.21,-2.4,8.11615888233178));
#11060=CARTESIAN_POINT('Ctrl Pts',(-0.21,-2.4,8.11615888233178));
#11061=CARTESIAN_POINT('Ctrl Pts',(-0.21,-2.37359906579625,8.11615888233178));
#11062=CARTESIAN_POINT('Ctrl Pts',(-0.20471752266132,-2.34545944463489,
8.11688606295397));
#11063=CARTESIAN_POINT('Ctrl Pts',(-0.183276841782292,-2.2937289476995,
8.11950502964782));
#11064=CARTESIAN_POINT('Ctrl Pts',(-0.167120287247804,-2.27013543914945,
8.12135816887013));
#11065=CARTESIAN_POINT('Ctrl Pts',(-0.129864750292352,-2.232879902194,8.12483075953278));
#11066=CARTESIAN_POINT('Ctrl Pts',(-0.106271159541076,-2.21672319916877,
8.12667690933009));
#11067=CARTESIAN_POINT('Ctrl Pts',(-0.0545403836274688,-2.1952824096556,
8.12927985626981));
#11068=CARTESIAN_POINT('Ctrl Pts',(-0.0264006657112965,-2.19,8.13));
#11069=CARTESIAN_POINT('Ctrl Pts',(0.0264006657112965,-2.19,8.13));
#11070=CARTESIAN_POINT('Ctrl Pts',(0.0545403836274689,-2.1952824096556,
8.12927985626981));
#11071=CARTESIAN_POINT('Ctrl Pts',(0.106271159541076,-2.21672319916877,
8.12667690933009));
#11072=CARTESIAN_POINT('Ctrl Pts',(0.129864750292352,-2.232879902194,8.12483075953278));
#11073=CARTESIAN_POINT('Ctrl Pts',(0.167120287247804,-2.27013543914945,
8.12135816887013));
#11074=CARTESIAN_POINT('Ctrl Pts',(0.183276841782292,-2.2937289476995,8.11950502964782));
#11075=CARTESIAN_POINT('Ctrl Pts',(0.20471752266132,-2.34545944463489,8.11688606295397));
#11076=CARTESIAN_POINT('Ctrl Pts',(0.21,-2.37359906579625,8.11615888233178));
#11077=CARTESIAN_POINT('Ctrl Pts',(0.21,-2.4,8.11615888233178));
#11078=CARTESIAN_POINT('',(-0.172988438920056,-2.28094119100208,7.52));
#11079=CARTESIAN_POINT('Origin',(0.,-2.4,7.52));
#11080=CARTESIAN_POINT('Ctrl Pts',(0.172988438920056,-2.28094119100209,
7.52));
#11081=CARTESIAN_POINT('Ctrl Pts',(0.165594865311314,-2.27019857760471,
7.52129192197638));
#11082=CARTESIAN_POINT('Ctrl Pts',(0.157297138725606,-2.26031229062726,
7.52265394943905));
#11083=CARTESIAN_POINT('Ctrl Pts',(0.129892073845076,-2.23290722574673,
7.5267480843909));
#11084=CARTESIAN_POINT('Ctrl Pts',(0.106330167759284,-2.21675794366705,
7.52969589327638));
#11085=CARTESIAN_POINT('Ctrl Pts',(0.0546129046324104,-2.19530220603509,
7.53385029472357));
#11086=CARTESIAN_POINT('Ctrl Pts',(0.0264512308298516,-2.19,7.535));
#11087=CARTESIAN_POINT('Ctrl Pts',(-0.0264512308298516,-2.19,7.535));
#11088=CARTESIAN_POINT('Ctrl Pts',(-0.0546129046324104,-2.19530220603509,
7.53385029472357));
#11089=CARTESIAN_POINT('Ctrl Pts',(-0.106330167759284,-2.21675794366705,
7.52969589327638));
#11090=CARTESIAN_POINT('Ctrl Pts',(-0.129892073845076,-2.23290722574673,
7.5267480843909));
#11091=CARTESIAN_POINT('Ctrl Pts',(-0.157297138725606,-2.26031229062726,
7.52265394943905));
#11092=CARTESIAN_POINT('Ctrl Pts',(-0.165594865311315,-2.27019857760471,
7.52129192197638));
#11093=CARTESIAN_POINT('Ctrl Pts',(-0.172988438920056,-2.28094119100208,
7.52));
#11094=CARTESIAN_POINT('Origin',(0.,-2.4,7.52));
#11095=CARTESIAN_POINT('',(-0.172988438920056,-3.6,7.52));
#11096=CARTESIAN_POINT('Origin',(0.,-2.9,6.53));
#11097=CARTESIAN_POINT('',(-1.6,-1.9,6.53));
#11098=CARTESIAN_POINT('Origin',(0.,-1.9,6.53));
#11099=CARTESIAN_POINT('',(-1.6,-2.9,6.53));
#11100=CARTESIAN_POINT('',(-1.6,-2.9,6.53));
#11101=CARTESIAN_POINT('Origin',(0.,-2.9,6.53));
#11102=CARTESIAN_POINT('Origin',(0.,-1.9,6.53));
#11103=CARTESIAN_POINT('',(-1.005,-1.9,6.53));
#11104=CARTESIAN_POINT('Origin',(0.,-1.9,6.53));
#11105=CARTESIAN_POINT('Origin',(0.,-3.6,6.53));
#11106=CARTESIAN_POINT('',(-1.005,-3.5,6.53));
#11107=CARTESIAN_POINT('Origin',(0.,-3.5,6.53));
#11108=CARTESIAN_POINT('',(-1.005,-3.6,6.53));
#11109=CARTESIAN_POINT('Origin',(4.,-3.5,6.53));
#11110=CARTESIAN_POINT('',(4.49999314610979,-3.5,6.52214602235346));
#11111=CARTESIAN_POINT('',(4.,-3.5,6.53));
#11112=CARTESIAN_POINT('',(4.49999314610979,-3.5,6.52214602235346));
#11113=CARTESIAN_POINT('',(4.49999314610979,-2.9,6.52214602235346));
#11114=CARTESIAN_POINT('',(4.49999314610979,-3.5,6.52214602235346));
#11115=CARTESIAN_POINT('',(4.,-2.9,6.53));
#11116=CARTESIAN_POINT('',(4.49999314610979,-2.9,6.52214602235346));
#11117=CARTESIAN_POINT('',(4.,-3.5,6.53));
#11118=CARTESIAN_POINT('Origin',(4.34869235694598,-3.5,7.68709756919613));
#11119=CARTESIAN_POINT('',(4.34869235694598,-3.5,7.68709756919613));
#11120=CARTESIAN_POINT('',(4.,-3.5,6.53));
#11121=CARTESIAN_POINT('',(4.34869235694598,-2.9,7.68709756919613));
#11122=CARTESIAN_POINT('',(4.,-2.9,6.53));
#11123=CARTESIAN_POINT('',(4.34869235694598,-3.5,7.68709756919613));
#11124=CARTESIAN_POINT('Origin',(3.86370330515627,-3.5,7.56527618041008));
#11125=CARTESIAN_POINT('',(3.86370330515627,-3.5,7.56527618041008));
#11126=CARTESIAN_POINT('',(4.34869235694598,-3.5,7.68709756919613));
#11127=CARTESIAN_POINT('',(3.86370330515627,-2.9,7.56527618041008));
#11128=CARTESIAN_POINT('',(4.34869235694598,-2.9,7.68709756919613));
#11129=CARTESIAN_POINT('',(3.86370330515627,-3.5,7.56527618041008));
#11130=CARTESIAN_POINT('Origin',(3.90103537021021,-3.5,8.77319482889224));
#11131=CARTESIAN_POINT('',(3.90103537021021,-3.5,8.77319482889224));
#11132=CARTESIAN_POINT('',(3.86370330515627,-3.5,7.56527618041008));
#11133=CARTESIAN_POINT('',(3.90103537021021,-2.9,8.77319482889224));
#11134=CARTESIAN_POINT('',(3.86370330515627,-2.9,7.56527618041008));
#11135=CARTESIAN_POINT('',(3.90103537021021,-3.5,8.77319482889224));
#11136=CARTESIAN_POINT('Origin',(3.46410161513775,-3.5,8.53));
#11137=CARTESIAN_POINT('',(3.46410161513775,-3.5,8.53));
#11138=CARTESIAN_POINT('',(3.90103537021021,-3.5,8.77319482889224));
#11139=CARTESIAN_POINT('',(3.46410161513775,-2.9,8.53));
#11140=CARTESIAN_POINT('',(3.90103537021021,-2.9,8.77319482889224));
#11141=CARTESIAN_POINT('',(3.46410161513775,-3.5,8.53));
#11142=CARTESIAN_POINT('Origin',(3.18752926976038,-3.5,9.70642206805406));
#11143=CARTESIAN_POINT('',(3.18752926976038,-3.5,9.70642206805406));
#11144=CARTESIAN_POINT('',(3.46410161513775,-3.5,8.53));
#11145=CARTESIAN_POINT('',(3.18752926976038,-2.9,9.70642206805406));
#11146=CARTESIAN_POINT('',(3.46410161513775,-2.9,8.53));
#11147=CARTESIAN_POINT('',(3.18752926976038,-3.5,9.70642206805406));
#11148=CARTESIAN_POINT('Origin',(2.82842712474619,-3.5,9.35842712474619));
#11149=CARTESIAN_POINT('',(2.82842712474619,-3.5,9.35842712474619));
#11150=CARTESIAN_POINT('',(3.18752926976038,-3.5,9.70642206805406));
#11151=CARTESIAN_POINT('',(2.82842712474619,-2.9,9.35842712474619));
#11152=CARTESIAN_POINT('',(3.18752926976038,-2.9,9.70642206805406));
#11153=CARTESIAN_POINT('',(2.82842712474619,-3.5,9.35842712474619));
#11154=CARTESIAN_POINT('Origin',(2.25679831721756,-3.5,10.4231813925637));
#11155=CARTESIAN_POINT('',(2.25679831721756,-3.5,10.4231813925637));
#11156=CARTESIAN_POINT('',(2.82842712474619,-3.5,9.35842712474619));
#11157=CARTESIAN_POINT('',(2.25679831721756,-2.9,10.4231813925637));
#11158=CARTESIAN_POINT('',(2.82842712474619,-2.9,9.35842712474619));
#11159=CARTESIAN_POINT('',(2.25679831721756,-3.5,10.4231813925637));
#11160=CARTESIAN_POINT('Origin',(2.,-3.5,9.99410161513775));
#11161=CARTESIAN_POINT('',(2.,-3.5,9.99410161513775));
#11162=CARTESIAN_POINT('',(2.25679831721756,-3.5,10.4231813925637));
#11163=CARTESIAN_POINT('',(2.,-2.9,9.99410161513775));
#11164=CARTESIAN_POINT('',(2.25679831721756,-2.9,10.4231813925637));
#11165=CARTESIAN_POINT('',(2.,-3.5,9.99410161513775));
#11166=CARTESIAN_POINT('Origin',(1.17227028889192,-3.5,10.8746268389565));
#11167=CARTESIAN_POINT('',(1.17227028889192,-3.5,10.8746268389565));
#11168=CARTESIAN_POINT('',(2.,-3.5,9.99410161513775));
#11169=CARTESIAN_POINT('',(1.17227028889192,-2.9,10.8746268389565));
#11170=CARTESIAN_POINT('',(2.,-2.9,9.99410161513775));
#11171=CARTESIAN_POINT('',(1.17227028889192,-3.5,10.8746268389565));
#11172=CARTESIAN_POINT('Origin',(1.03527618041008,-3.5,10.3937033051563));
#11173=CARTESIAN_POINT('',(1.03527618041008,-3.5,10.3937033051563));
#11174=CARTESIAN_POINT('',(1.17227028889192,-3.5,10.8746268389565));
#11175=CARTESIAN_POINT('',(1.03527618041008,-2.9,10.3937033051563));
#11176=CARTESIAN_POINT('',(1.17227028889192,-2.9,10.8746268389565));
#11177=CARTESIAN_POINT('',(1.03527618041008,-3.5,10.3937033051563));
#11178=CARTESIAN_POINT('Origin',(0.00785397764654228,-3.5,11.0299931461098));
#11179=CARTESIAN_POINT('',(0.00785397764654218,-3.5,11.0299931461098));
#11180=CARTESIAN_POINT('',(1.03527618041008,-3.5,10.3937033051563));
#11181=CARTESIAN_POINT('',(0.00785397764654228,-2.9,11.0299931461098));
#11182=CARTESIAN_POINT('',(1.03527618041008,-2.9,10.3937033051563));
#11183=CARTESIAN_POINT('',(0.00785397764654218,-3.5,11.0299931461098));
#11184=CARTESIAN_POINT('Origin',(2.4459601011273E-16,-3.5,10.53));
#11185=CARTESIAN_POINT('',(2.44929359829471E-16,-3.5,10.53));
#11186=CARTESIAN_POINT('',(0.00785397764654218,-3.5,11.0299931461098));
#11187=CARTESIAN_POINT('',(4.44089209850063E-16,-2.9,10.53));
#11188=CARTESIAN_POINT('',(0.00785397764654218,-2.9,11.0299931461098));
#11189=CARTESIAN_POINT('',(2.44929359829471E-16,-3.5,10.53));
#11190=CARTESIAN_POINT('Origin',(-1.15709756919613,-3.5,10.878692356946));
#11191=CARTESIAN_POINT('',(-1.15709756919613,-3.5,10.878692356946));
#11192=CARTESIAN_POINT('',(2.44929359829471E-16,-3.5,10.53));
#11193=CARTESIAN_POINT('',(-1.15709756919613,-2.9,10.878692356946));
#11194=CARTESIAN_POINT('',(2.44929359829471E-16,-2.9,10.53));
#11195=CARTESIAN_POINT('',(-1.15709756919613,-3.5,10.878692356946));
#11196=CARTESIAN_POINT('Origin',(-1.03527618041008,-3.5,10.3937033051563));
#11197=CARTESIAN_POINT('',(-1.03527618041008,-3.5,10.3937033051563));
#11198=CARTESIAN_POINT('',(-1.15709756919613,-3.5,10.878692356946));
#11199=CARTESIAN_POINT('',(-1.03527618041008,-2.9,10.3937033051563));
#11200=CARTESIAN_POINT('',(-1.15709756919613,-2.9,10.878692356946));
#11201=CARTESIAN_POINT('',(-1.03527618041008,-3.5,10.3937033051563));
#11202=CARTESIAN_POINT('Origin',(-2.24319482889224,-3.5,10.4310353702102));
#11203=CARTESIAN_POINT('',(-2.24319482889224,-3.5,10.4310353702102));
#11204=CARTESIAN_POINT('',(-1.03527618041008,-3.5,10.3937033051563));
#11205=CARTESIAN_POINT('',(-2.24319482889224,-2.9,10.4310353702102));
#11206=CARTESIAN_POINT('',(-1.03527618041008,-2.9,10.3937033051563));
#11207=CARTESIAN_POINT('',(-2.24319482889224,-3.5,10.4310353702102));
#11208=CARTESIAN_POINT('Origin',(-2.,-3.5,9.99410161513775));
#11209=CARTESIAN_POINT('',(-2.,-3.5,9.99410161513775));
#11210=CARTESIAN_POINT('',(-2.24319482889224,-3.5,10.4310353702102));
#11211=CARTESIAN_POINT('',(-2.,-2.9,9.99410161513775));
#11212=CARTESIAN_POINT('',(-2.24319482889224,-2.9,10.4310353702102));
#11213=CARTESIAN_POINT('',(-2.,-3.5,9.99410161513775));
#11214=CARTESIAN_POINT('Origin',(-3.17642206805406,-3.5,9.71752926976038));
#11215=CARTESIAN_POINT('',(-3.17642206805406,-3.5,9.71752926976038));
#11216=CARTESIAN_POINT('',(-2.,-3.5,9.99410161513775));
#11217=CARTESIAN_POINT('',(-3.17642206805406,-2.9,9.71752926976038));
#11218=CARTESIAN_POINT('',(-2.,-2.9,9.99410161513775));
#11219=CARTESIAN_POINT('',(-3.17642206805406,-3.5,9.71752926976038));
#11220=CARTESIAN_POINT('Origin',(-2.82842712474619,-3.5,9.35842712474619));
#11221=CARTESIAN_POINT('',(-2.82842712474619,-3.5,9.35842712474619));
#11222=CARTESIAN_POINT('',(-3.17642206805406,-3.5,9.71752926976038));
#11223=CARTESIAN_POINT('',(-2.82842712474619,-2.9,9.35842712474619));
#11224=CARTESIAN_POINT('',(-3.17642206805406,-2.9,9.71752926976038));
#11225=CARTESIAN_POINT('',(-2.82842712474619,-3.5,9.35842712474619));
#11226=CARTESIAN_POINT('Origin',(-3.89318139256367,-3.5,8.78679831721756));
#11227=CARTESIAN_POINT('',(-3.89318139256367,-3.5,8.78679831721756));
#11228=CARTESIAN_POINT('',(-2.82842712474619,-3.5,9.35842712474619));
#11229=CARTESIAN_POINT('',(-3.89318139256367,-2.9,8.78679831721756));
#11230=CARTESIAN_POINT('',(-2.82842712474619,-2.9,9.35842712474619));
#11231=CARTESIAN_POINT('',(-3.89318139256367,-3.5,8.78679831721756));
#11232=CARTESIAN_POINT('Origin',(-3.46410161513775,-3.5,8.53));
#11233=CARTESIAN_POINT('',(-3.46410161513775,-3.5,8.53));
#11234=CARTESIAN_POINT('',(-3.89318139256367,-3.5,8.78679831721756));
#11235=CARTESIAN_POINT('',(-3.46410161513775,-2.9,8.53));
#11236=CARTESIAN_POINT('',(-3.89318139256367,-2.9,8.78679831721756));
#11237=CARTESIAN_POINT('',(-3.46410161513775,-3.5,8.53));
#11238=CARTESIAN_POINT('Origin',(-4.34462683895651,-3.5,7.70227028889192));
#11239=CARTESIAN_POINT('',(-4.34462683895651,-3.5,7.70227028889192));
#11240=CARTESIAN_POINT('',(-3.46410161513775,-3.5,8.53));
#11241=CARTESIAN_POINT('',(-4.34462683895651,-2.9,7.70227028889192));
#11242=CARTESIAN_POINT('',(-3.46410161513775,-2.9,8.53));
#11243=CARTESIAN_POINT('',(-4.34462683895651,-3.5,7.70227028889192));
#11244=CARTESIAN_POINT('Origin',(-3.86370330515627,-3.5,7.56527618041008));
#11245=CARTESIAN_POINT('',(-3.86370330515627,-3.5,7.56527618041008));
#11246=CARTESIAN_POINT('',(-4.34462683895651,-3.5,7.70227028889192));
#11247=CARTESIAN_POINT('',(-3.86370330515627,-2.9,7.56527618041008));
#11248=CARTESIAN_POINT('',(-4.34462683895651,-2.9,7.70227028889192));
#11249=CARTESIAN_POINT('',(-3.86370330515627,-3.5,7.56527618041008));
#11250=CARTESIAN_POINT('Origin',(-4.49999314610979,-3.5,6.53785397764654));
#11251=CARTESIAN_POINT('',(-4.49999314610979,-3.5,6.53785397764654));
#11252=CARTESIAN_POINT('',(-3.86370330515627,-3.5,7.56527618041008));
#11253=CARTESIAN_POINT('',(-4.49999314610979,-2.9,6.53785397764654));
#11254=CARTESIAN_POINT('',(-3.86370330515627,-2.9,7.56527618041008));
#11255=CARTESIAN_POINT('',(-4.49999314610979,-3.5,6.53785397764654));
#11256=CARTESIAN_POINT('Origin',(-4.,-3.5,6.53));
#11257=CARTESIAN_POINT('',(-4.,-3.5,6.53));
#11258=CARTESIAN_POINT('',(-4.49999314610979,-3.5,6.53785397764654));
#11259=CARTESIAN_POINT('',(-4.,-2.9,6.53));
#11260=CARTESIAN_POINT('',(-4.49999314610979,-2.9,6.53785397764654));
#11261=CARTESIAN_POINT('',(-4.,-3.5,6.53));
#11262=CARTESIAN_POINT('Origin',(-4.34869235694598,-3.5,5.37290243080387));
#11263=CARTESIAN_POINT('',(-4.34869235694598,-3.5,5.37290243080387));
#11264=CARTESIAN_POINT('',(-4.,-3.5,6.53));
#11265=CARTESIAN_POINT('',(-4.34869235694598,-2.9,5.37290243080387));
#11266=CARTESIAN_POINT('',(-4.,-2.9,6.53));
#11267=CARTESIAN_POINT('',(-4.34869235694598,-3.5,5.37290243080387));
#11268=CARTESIAN_POINT('Origin',(-3.86370330515627,-3.5,5.49472381958992));
#11269=CARTESIAN_POINT('',(-3.86370330515627,-3.5,5.49472381958992));
#11270=CARTESIAN_POINT('',(-4.34869235694598,-3.5,5.37290243080387));
#11271=CARTESIAN_POINT('',(-3.86370330515627,-2.9,5.49472381958992));
#11272=CARTESIAN_POINT('',(-4.34869235694598,-2.9,5.37290243080387));
#11273=CARTESIAN_POINT('',(-3.86370330515627,-3.5,5.49472381958992));
#11274=CARTESIAN_POINT('Origin',(-3.90103537021021,-3.5,4.28680517110776));
#11275=CARTESIAN_POINT('',(-3.90103537021021,-3.5,4.28680517110776));
#11276=CARTESIAN_POINT('',(-3.86370330515627,-3.5,5.49472381958992));
#11277=CARTESIAN_POINT('',(-3.90103537021021,-2.9,4.28680517110776));
#11278=CARTESIAN_POINT('',(-3.86370330515627,-2.9,5.49472381958992));
#11279=CARTESIAN_POINT('',(-3.90103537021021,-3.5,4.28680517110776));
#11280=CARTESIAN_POINT('Origin',(-3.46410161513775,-3.5,4.53));
#11281=CARTESIAN_POINT('',(-3.46410161513775,-3.5,4.53));
#11282=CARTESIAN_POINT('',(-3.90103537021021,-3.5,4.28680517110776));
#11283=CARTESIAN_POINT('',(-3.46410161513775,-2.9,4.53));
#11284=CARTESIAN_POINT('',(-3.90103537021021,-2.9,4.28680517110776));
#11285=CARTESIAN_POINT('',(-3.46410161513775,-3.5,4.53));
#11286=CARTESIAN_POINT('Origin',(-3.18752926976038,-3.5,3.35357793194594));
#11287=CARTESIAN_POINT('',(-3.18752926976038,-3.5,3.35357793194594));
#11288=CARTESIAN_POINT('',(-3.46410161513775,-3.5,4.53));
#11289=CARTESIAN_POINT('',(-3.18752926976038,-2.9,3.35357793194594));
#11290=CARTESIAN_POINT('',(-3.46410161513775,-2.9,4.53));
#11291=CARTESIAN_POINT('',(-3.18752926976038,-3.5,3.35357793194594));
#11292=CARTESIAN_POINT('Origin',(-2.82842712474619,-3.5,3.70157287525381));
#11293=CARTESIAN_POINT('',(-2.82842712474619,-3.5,3.70157287525381));
#11294=CARTESIAN_POINT('',(-3.18752926976038,-3.5,3.35357793194594));
#11295=CARTESIAN_POINT('',(-2.82842712474619,-2.9,3.70157287525381));
#11296=CARTESIAN_POINT('',(-3.18752926976038,-2.9,3.35357793194594));
#11297=CARTESIAN_POINT('',(-2.82842712474619,-3.5,3.70157287525381));
#11298=CARTESIAN_POINT('Origin',(-2.25679831721756,-3.5,2.63681860743633));
#11299=CARTESIAN_POINT('',(-2.25679831721756,-3.5,2.63681860743633));
#11300=CARTESIAN_POINT('',(-2.82842712474619,-3.5,3.70157287525381));
#11301=CARTESIAN_POINT('',(-2.25679831721756,-2.9,2.63681860743633));
#11302=CARTESIAN_POINT('',(-2.82842712474619,-2.9,3.70157287525381));
#11303=CARTESIAN_POINT('',(-2.25679831721756,-3.5,2.63681860743633));
#11304=CARTESIAN_POINT('Origin',(-2.,-3.5,3.06589838486225));
#11305=CARTESIAN_POINT('',(-2.,-3.5,3.06589838486225));
#11306=CARTESIAN_POINT('',(-2.25679831721756,-3.5,2.63681860743633));
#11307=CARTESIAN_POINT('',(-2.,-2.9,3.06589838486225));
#11308=CARTESIAN_POINT('',(-2.25679831721756,-2.9,2.63681860743633));
#11309=CARTESIAN_POINT('',(-2.,-3.5,3.06589838486225));
#11310=CARTESIAN_POINT('Origin',(-1.17227028889192,-3.5,2.18537316104349));
#11311=CARTESIAN_POINT('',(-1.17227028889192,-3.5,2.18537316104349));
#11312=CARTESIAN_POINT('',(-2.,-3.5,3.06589838486225));
#11313=CARTESIAN_POINT('',(-1.17227028889192,-2.9,2.18537316104349));
#11314=CARTESIAN_POINT('',(-2.,-2.9,3.06589838486225));
#11315=CARTESIAN_POINT('',(-1.17227028889192,-3.5,2.18537316104349));
#11316=CARTESIAN_POINT('Origin',(-1.03527618041008,-3.5,2.66629669484373));
#11317=CARTESIAN_POINT('',(-1.03527618041008,-3.5,2.66629669484373));
#11318=CARTESIAN_POINT('',(-1.17227028889192,-3.5,2.18537316104349));
#11319=CARTESIAN_POINT('',(-1.03527618041008,-2.9,2.66629669484373));
#11320=CARTESIAN_POINT('',(-1.17227028889192,-2.9,2.18537316104349));
#11321=CARTESIAN_POINT('',(-1.03527618041008,-3.5,2.66629669484373));
#11322=CARTESIAN_POINT('Origin',(-0.00785397764654272,-3.5,2.03000685389021));
#11323=CARTESIAN_POINT('',(-0.00785397764654273,-3.5,2.03000685389021));
#11324=CARTESIAN_POINT('',(-1.03527618041008,-3.5,2.66629669484373));
#11325=CARTESIAN_POINT('',(-0.00785397764654272,-2.9,2.03000685389021));
#11326=CARTESIAN_POINT('',(-1.03527618041008,-2.9,2.66629669484373));
#11327=CARTESIAN_POINT('',(-0.00785397764654273,-3.5,2.03000685389021));
#11328=CARTESIAN_POINT('Origin',(-7.35522753814166E-16,-3.5,2.53));
#11329=CARTESIAN_POINT('',(-7.34788079488412E-16,-3.5,2.53));
#11330=CARTESIAN_POINT('',(-0.00785397764654273,-3.5,2.03000685389021));
#11331=CARTESIAN_POINT('',(-8.88178419700125E-16,-2.9,2.53));
#11332=CARTESIAN_POINT('',(-0.00785397764654273,-2.9,2.03000685389021));
#11333=CARTESIAN_POINT('',(-7.34788079488412E-16,-3.5,2.53));
#11334=CARTESIAN_POINT('Origin',(1.15709756919613,-3.5,2.18130764305402));
#11335=CARTESIAN_POINT('',(1.15709756919613,-3.5,2.18130764305402));
#11336=CARTESIAN_POINT('',(-7.34788079488412E-16,-3.5,2.53));
#11337=CARTESIAN_POINT('',(1.15709756919613,-2.9,2.18130764305402));
#11338=CARTESIAN_POINT('',(-7.34788079488412E-16,-2.9,2.53));
#11339=CARTESIAN_POINT('',(1.15709756919613,-3.5,2.18130764305402));
#11340=CARTESIAN_POINT('Origin',(1.03527618041008,-3.5,2.66629669484373));
#11341=CARTESIAN_POINT('',(1.03527618041008,-3.5,2.66629669484373));
#11342=CARTESIAN_POINT('',(1.15709756919613,-3.5,2.18130764305402));
#11343=CARTESIAN_POINT('',(1.03527618041008,-2.9,2.66629669484373));
#11344=CARTESIAN_POINT('',(1.15709756919613,-2.9,2.18130764305402));
#11345=CARTESIAN_POINT('',(1.03527618041008,-3.5,2.66629669484373));
#11346=CARTESIAN_POINT('Origin',(2.24319482889223,-3.5,2.62896462978979));
#11347=CARTESIAN_POINT('',(2.24319482889223,-3.5,2.62896462978979));
#11348=CARTESIAN_POINT('',(1.03527618041008,-3.5,2.66629669484373));
#11349=CARTESIAN_POINT('',(2.24319482889223,-2.9,2.62896462978979));
#11350=CARTESIAN_POINT('',(1.03527618041008,-2.9,2.66629669484373));
#11351=CARTESIAN_POINT('',(2.24319482889223,-3.5,2.62896462978979));
#11352=CARTESIAN_POINT('Origin',(2.,-3.5,3.06589838486225));
#11353=CARTESIAN_POINT('',(2.,-3.5,3.06589838486225));
#11354=CARTESIAN_POINT('',(2.24319482889223,-3.5,2.62896462978979));
#11355=CARTESIAN_POINT('',(2.,-2.9,3.06589838486225));
#11356=CARTESIAN_POINT('',(2.24319482889223,-2.9,2.62896462978979));
#11357=CARTESIAN_POINT('',(2.,-3.5,3.06589838486225));
#11358=CARTESIAN_POINT('Origin',(3.17642206805406,-3.5,3.34247073023962));
#11359=CARTESIAN_POINT('',(3.17642206805406,-3.5,3.34247073023962));
#11360=CARTESIAN_POINT('',(2.,-3.5,3.06589838486225));
#11361=CARTESIAN_POINT('',(3.17642206805406,-2.9,3.34247073023962));
#11362=CARTESIAN_POINT('',(2.,-2.9,3.06589838486225));
#11363=CARTESIAN_POINT('',(3.17642206805406,-3.5,3.34247073023962));
#11364=CARTESIAN_POINT('Origin',(2.82842712474619,-3.5,3.70157287525381));
#11365=CARTESIAN_POINT('',(2.82842712474619,-3.5,3.70157287525381));
#11366=CARTESIAN_POINT('',(3.17642206805406,-3.5,3.34247073023962));
#11367=CARTESIAN_POINT('',(2.82842712474619,-2.9,3.70157287525381));
#11368=CARTESIAN_POINT('',(3.17642206805406,-2.9,3.34247073023962));
#11369=CARTESIAN_POINT('',(2.82842712474619,-3.5,3.70157287525381));
#11370=CARTESIAN_POINT('Origin',(3.89318139256367,-3.5,4.27320168278244));
#11371=CARTESIAN_POINT('',(3.89318139256367,-3.5,4.27320168278244));
#11372=CARTESIAN_POINT('',(2.82842712474619,-3.5,3.70157287525381));
#11373=CARTESIAN_POINT('',(3.89318139256367,-2.9,4.27320168278244));
#11374=CARTESIAN_POINT('',(2.82842712474619,-2.9,3.70157287525381));
#11375=CARTESIAN_POINT('',(3.89318139256367,-3.5,4.27320168278244));
#11376=CARTESIAN_POINT('Origin',(3.46410161513775,-3.5,4.53));
#11377=CARTESIAN_POINT('',(3.46410161513775,-3.5,4.53));
#11378=CARTESIAN_POINT('',(3.89318139256367,-3.5,4.27320168278244));
#11379=CARTESIAN_POINT('',(3.46410161513775,-2.9,4.53));
#11380=CARTESIAN_POINT('',(3.89318139256367,-2.9,4.27320168278244));
#11381=CARTESIAN_POINT('',(3.46410161513775,-3.5,4.53));
#11382=CARTESIAN_POINT('Origin',(4.34462683895651,-3.5,5.35772971110808));
#11383=CARTESIAN_POINT('',(4.34462683895651,-3.5,5.35772971110808));
#11384=CARTESIAN_POINT('',(3.46410161513775,-3.5,4.53));
#11385=CARTESIAN_POINT('',(4.34462683895651,-2.9,5.35772971110808));
#11386=CARTESIAN_POINT('',(3.46410161513775,-2.9,4.53));
#11387=CARTESIAN_POINT('',(4.34462683895651,-3.5,5.35772971110808));
#11388=CARTESIAN_POINT('Origin',(3.86370330515627,-3.5,5.49472381958992));
#11389=CARTESIAN_POINT('',(3.86370330515627,-3.5,5.49472381958992));
#11390=CARTESIAN_POINT('',(4.34462683895651,-3.5,5.35772971110808));
#11391=CARTESIAN_POINT('',(3.86370330515627,-2.9,5.49472381958992));
#11392=CARTESIAN_POINT('',(4.34462683895651,-2.9,5.35772971110808));
#11393=CARTESIAN_POINT('',(3.86370330515627,-3.5,5.49472381958992));
#11394=CARTESIAN_POINT('Origin',(4.49999314610979,-3.5,6.52214602235346));
#11395=CARTESIAN_POINT('',(3.86370330515627,-3.5,5.49472381958992));
#11396=CARTESIAN_POINT('',(3.86370330515627,-2.9,5.49472381958992));
#11397=CARTESIAN_POINT('Origin',(0.,-2.9,6.53));
#11398=CARTESIAN_POINT('Origin',(0.,-3.5,6.53));
#11754=UNCERTAINTY_MEASURE_WITH_UNIT(LENGTH_MEASURE(0.001),#11802,
'DISTANCE_ACCURACY_VALUE',
'Maximum model space distance between geometric entities at asserted c
onnectivities');
#11761=UNCERTAINTY_MEASURE_WITH_UNIT(LENGTH_MEASURE(0.001),#11802,
'DISTANCE_ACCURACY_VALUE',
'Maximum model space distance between geometric entities at asserted c
onnectivities');
#11794=(
GEOMETRIC_REPRESENTATION_CONTEXT(3)
GLOBAL_UNCERTAINTY_ASSIGNED_CONTEXT((#11754))
GLOBAL_UNIT_ASSIGNED_CONTEXT((#11802,#11804,#11805))
REPRESENTATION_CONTEXT('','3D')
);
#11801=(
GEOMETRIC_REPRESENTATION_CONTEXT(3)
GLOBAL_UNCERTAINTY_ASSIGNED_CONTEXT((#11761))
GLOBAL_UNIT_ASSIGNED_CONTEXT((#11802,#11804,#11805))
REPRESENTATION_CONTEXT('','3D')
);
#11802=(
LENGTH_UNIT()
NAMED_UNIT(*)
SI_UNIT(.CENTI.,.METRE.)
);
#11804=(
NAMED_UNIT(*)
PLANE_ANGLE_UNIT()
SI_UNIT($,.RADIAN.)
);
#11805=(
NAMED_UNIT(*)
SI_UNIT($,.STERADIAN.)
SOLID_ANGLE_UNIT()
);
#11838=SHAPE_DEFINITION_REPRESENTATION(#11879,#11977);
#11879=PRODUCT_DEFINITION_SHAPE('',$,#12017);
#11977=SHAPE_REPRESENTATION('',(#7143),#11794);
#11984=PRODUCT_DEFINITION_CONTEXT('part definition',#12103,'design');
#12017=PRODUCT_DEFINITION('Ratchet wheel','Ratchet wheel',#12056,#11984);
#12056=PRODUCT_DEFINITION_FORMATION('',$,#12137);
#12103=APPLICATION_CONTEXT(
'Core Data for Automotive Mechanical Design Process');
#12104=PRODUCT_CONTEXT('part definition',#12103,'mechanical');
#12137=PRODUCT('Ratchet wheel','Ratchet wheel','Ratchet wheel',(#12104));
#12200=COLOUR_RGB('Sky Blue',0.24,0.69,0.87);
#12201=FILL_AREA_STYLE_COLOUR('',#12200);
#12202=FILL_AREA_STYLE('',(#12201));
#12203=SURFACE_STYLE_FILL_AREA(#12202);
#12204=SURFACE_SIDE_STYLE('',(#12203));
#12205=SURFACE_STYLE_USAGE(.BOTH.,#12204);
#12206=PRESENTATION_STYLE_ASSIGNMENT((#12205));
ENDSEC;
END-ISO-10303-21;
